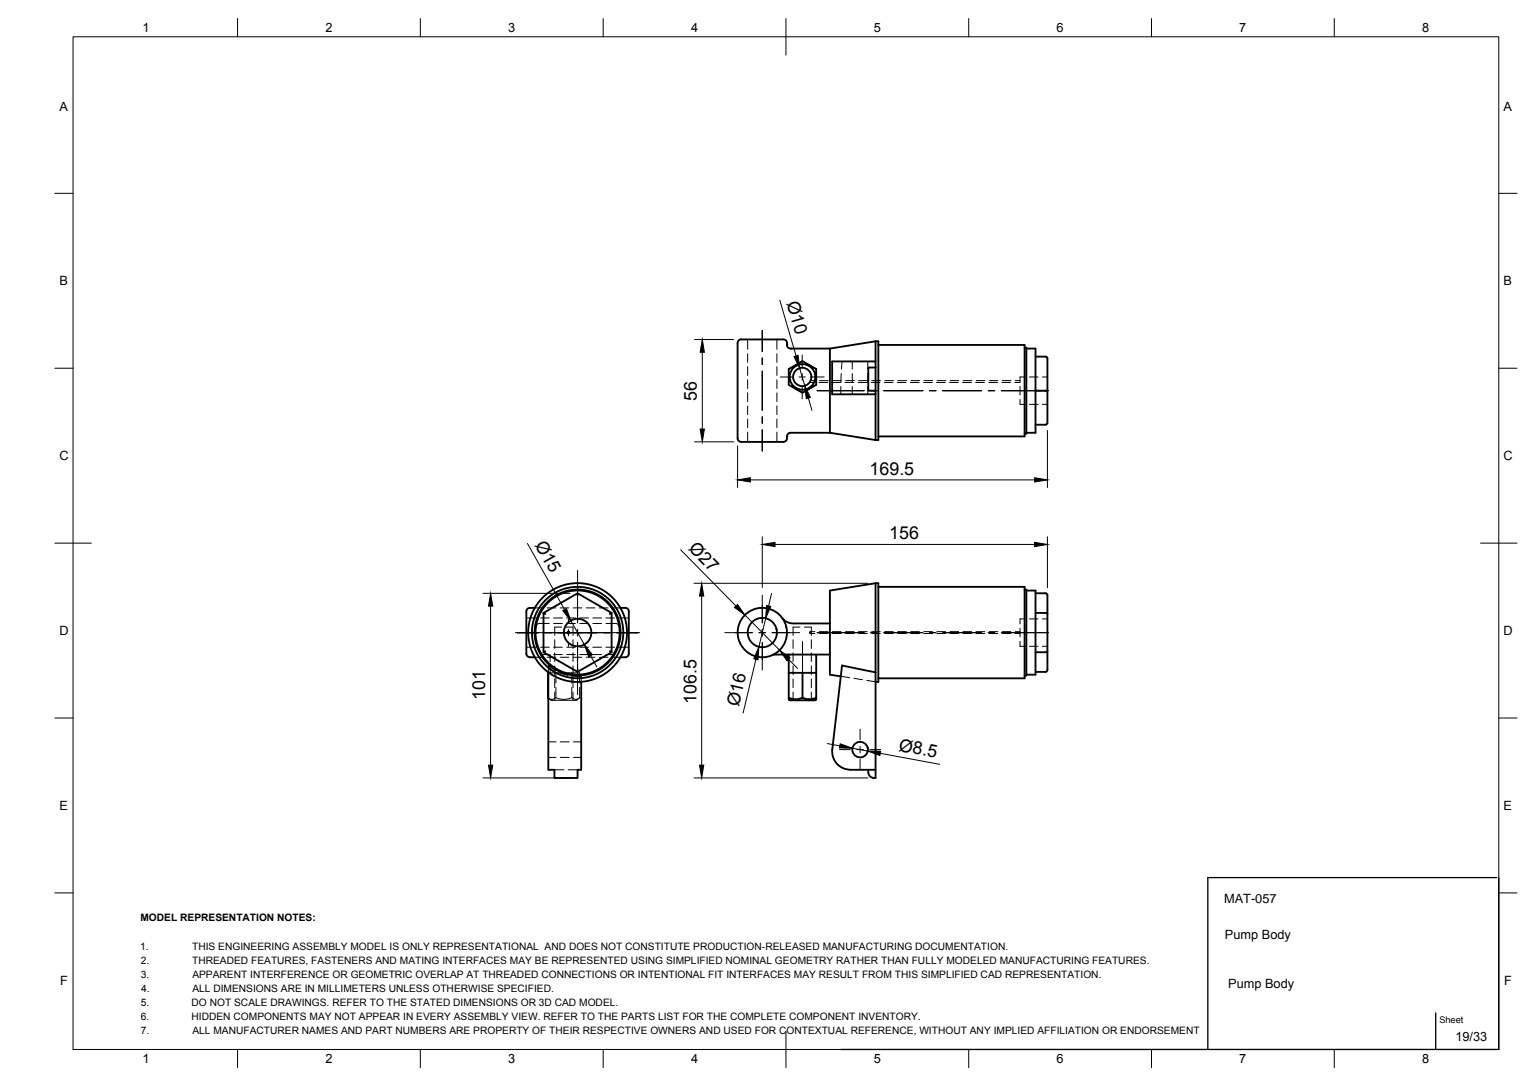
ISO-10303-21;
HEADER;
/* Generated by software containing ST-Developer
 * from STEP Tools, Inc. (www.steptools.com) 
 */

FILE_DESCRIPTION(
/* description */ ('STEP AP214', 'CAx-IF Rec.Pracs.---Representation and Presentation of Product Manufa
cturing Information (PMI)---4.0---2014-10-13'),
/* implementation_level */ '2;1');

FILE_NAME(
/* name */ 'Pump Body.step',
/* time_stamp */ '2026-10-28T23:34:22+01:00',
/* author */ (''),
/* organization */ (''),
/* preprocessor_version */ 'ST-DEVELOPER v20.2',
/* originating_system */ 'Autodesk Translation Framework v15.17.0.0',
/* authorisation */ '');

FILE_SCHEMA (('AP242_MANAGED_MODEL_BASED_3D_ENGINEERING_MIM_LF { 1 0 10303 442 2 1 4 }'));
ENDSEC;

DATA;
#10=MECHANICAL_DESIGN_GEOMETRIC_PRESENTATION_REPRESENTATION('',(#259),#27807);
#35=(
BOUNDED_CURVE()
B_SPLINE_CURVE(2,(#19569,#19570,#19571),.UNSPECIFIED.,.F.,.F.)
B_SPLINE_CURVE_WITH_KNOTS((3,3),(3.35159796330511,5.11240655080017),
 .UNSPECIFIED.)
CURVE()
GEOMETRIC_REPRESENTATION_ITEM()
RATIONAL_B_SPLINE_CURVE((1.02178867577785,1.02219740253536,1.01702175780134))
REPRESENTATION_ITEM('')
);
#213=SHAPE_REPRESENTATION_RELATIONSHIP('SRR','None',#27910,#235);
#235=ADVANCED_BREP_SHAPE_REPRESENTATION('',(#288),#27790);
#259=STYLED_ITEM('',(#28056),#288);
#288=MANIFOLD_SOLID_BREP('Body1',#12035);
#310=(
BOUNDED_SURFACE()
B_SPLINE_SURFACE(3,2,((#20429,#20430,#20431),(#20432,#20433,#20434),(#20435,
#20436,#20437),(#20438,#20439,#20440),(#20441,#20442,#20443),(#20444,#20445,
#20446),(#20447,#20448,#20449),(#20450,#20451,#20452),(#20453,#20454,#20455),
(#20456,#20457,#20458),(#20459,#20460,#20461),(#20462,#20463,#20464),(#20465,
#20466,#20467),(#20468,#20469,#20470)),.UNSPECIFIED.,.F.,.F.,.F.)
B_SPLINE_SURFACE_WITH_KNOTS((4,2,2,2,2,2,4),(3,3),(2.29850860566927E-17,
0.00228352475280831,0.00342528712921246,0.00456704950561661,0.00570881188202075,
0.0068505742584249,0.00913409901123319),(0.,1.),.UNSPECIFIED.)
GEOMETRIC_REPRESENTATION_ITEM()
RATIONAL_B_SPLINE_SURFACE(((1.,0.755928946018453,1.),(1.,0.755919473251654,
1.),(1.,0.756953933195057,1.),(1.,0.759617125008032,1.),(1.,0.760694585385831,
1.),(1.,0.763054974489942,1.),(1.,0.764326129773376,1.),(1.,0.766864760301965,
1.),(1.,0.768132555731698,1.),(1.,0.770457118175421,1.),(1.,0.77151907153067,
1.),(1.,0.773976852479458,1.),(1.,0.774660609303815,1.),(1.,0.773601014837504,
1.)))
REPRESENTATION_ITEM('')
SURFACE()
);
#311=(
BOUNDED_SURFACE()
B_SPLINE_SURFACE(3,2,((#20547,#20548,#20549),(#20550,#20551,#20552),(#20553,
#20554,#20555),(#20556,#20557,#20558),(#20559,#20560,#20561),(#20562,#20563,
#20564),(#20565,#20566,#20567),(#20568,#20569,#20570),(#20571,#20572,#20573),
(#20574,#20575,#20576),(#20577,#20578,#20579),(#20580,#20581,#20582)),
 .UNSPECIFIED.,.F.,.F.,.F.)
B_SPLINE_SURFACE_WITH_KNOTS((4,2,2,2,2,4),(3,3),(-8.67361737988404E-18,
0.0020019127931021,0.00400382558620421,0.00500478198275526,0.00600573837930632,
0.00800765117240843),(0.,1.),.UNSPECIFIED.)
GEOMETRIC_REPRESENTATION_ITEM()
RATIONAL_B_SPLINE_SURFACE(((1.,0.720245417210284,1.),(1.,0.745456109699134,
1.),(1.,0.776939871169668,1.),(1.,0.843085998617067,1.),(1.,0.876043548544159,
1.),(1.,0.919062364122798,1.),(1.,0.932399541573303,1.),(1.,0.955903426154376,
1.),(1.,0.966062375399352,1.),(1.,0.990944979726916,1.),(1.,1.00003808704948,
1.),(1.,1.,1.)))
REPRESENTATION_ITEM('')
SURFACE()
);
#312=(
BOUNDED_SURFACE()
B_SPLINE_SURFACE(3,2,((#20584,#20585,#20586),(#20587,#20588,#20589),(#20590,
#20591,#20592),(#20593,#20594,#20595),(#20596,#20597,#20598),(#20599,#20600,
#20601),(#20602,#20603,#20604),(#20605,#20606,#20607),(#20608,#20609,#20610),
(#20611,#20612,#20613),(#20614,#20615,#20616),(#20617,#20618,#20619),(#20620,
#20621,#20622),(#20623,#20624,#20625),(#20626,#20627,#20628),(#20629,#20630,
#20631),(#20632,#20633,#20634),(#20635,#20636,#20637)),.UNSPECIFIED.,.F.,
 .F.,.F.)
B_SPLINE_SURFACE_WITH_KNOTS((4,2,2,2,2,2,2,2,4),(3,3),(0.0465879948739151,
0.0488019169422094,0.0499088779763565,0.0510158390105036,0.0532297610787979,
0.054336722112945,0.0554436831470922,0.0598715272836807,0.0642993714202692),
(0.,1.),.UNSPECIFIED.)
GEOMETRIC_REPRESENTATION_ITEM()
RATIONAL_B_SPLINE_SURFACE(((1.,0.720245417210284,1.),(1.,0.715430366769561,
1.),(1.,0.711757488391321,1.),(1.,0.708436125845732,1.),(1.,0.707701704610594,
1.),(1.,0.706997400069913,1.),(1.,0.70703042471459,1.),(1.,0.708269366538293,
1.),(1.,0.710603787640094,1.),(1.,0.716102617085572,1.),(1.,0.718267907422322,
1.),(1.,0.723213640275136,1.),(1.,0.726004552476763,1.),(1.,0.741243869654837,
1.),(1.,0.757174433729962,1.),(1.,0.791690080044701,1.),(1.,0.809643404127687,
1.),(1.,0.826358787974886,1.)))
REPRESENTATION_ITEM('')
SURFACE()
);
#313=(
BOUNDED_SURFACE()
B_SPLINE_SURFACE(3,2,((#20719,#20720,#20721),(#20722,#20723,#20724),(#20725,
#20726,#20727),(#20728,#20729,#20730),(#20731,#20732,#20733),(#20734,#20735,
#20736),(#20737,#20738,#20739),(#20740,#20741,#20742),(#20743,#20744,#20745),
(#20746,#20747,#20748),(#20749,#20750,#20751),(#20752,#20753,#20754),(#20755,
#20756,#20757),(#20758,#20759,#20760),(#20761,#20762,#20763),(#20764,#20765,
#20766)),.UNSPECIFIED.,.F.,.F.,.F.)
B_SPLINE_SURFACE_WITH_KNOTS((4,2,2,2,2,2,2,4),(3,3),(0.00572874702066893,
0.00641318489301232,0.00709762276535571,0.00778206063769909,0.00846649851004248,
0.00915093638238587,0.00983537425472925,0.011204249999416),(0.,1.),
 .UNSPECIFIED.)
GEOMETRIC_REPRESENTATION_ITEM()
RATIONAL_B_SPLINE_SURFACE(((1.,0.975506485486288,1.),(1.,0.975513146220073,
1.),(1.,0.973968479244861,1.),(1.,0.968411518445162,1.),(1.,0.964542733059259,
1.),(1.,0.955226889333692,1.),(1.,0.949822152420214,1.),(1.,0.938073995978702,
1.),(1.,0.931687255706716,1.),(1.,0.918003026598242,1.),(1.,0.91068796451963,
1.),(1.,0.895477555573003,1.),(1.,0.887548913896672,1.),(1.,0.862850245396308,
1.),(1.,0.845167627106926,1.),(1.,0.826358787974873,1.)))
REPRESENTATION_ITEM('')
SURFACE()
);
#314=(
BOUNDED_SURFACE()
B_SPLINE_SURFACE(3,2,((#20852,#20853,#20854),(#20855,#20856,#20857),(#20858,
#20859,#20860),(#20861,#20862,#20863),(#20864,#20865,#20866),(#20867,#20868,
#20869),(#20870,#20871,#20872),(#20873,#20874,#20875),(#20876,#20877,#20878),
(#20879,#20880,#20881),(#20882,#20883,#20884),(#20885,#20886,#20887),(#20888,
#20889,#20890),(#20891,#20892,#20893)),.UNSPECIFIED.,.F.,.F.,.F.)
B_SPLINE_SURFACE_WITH_KNOTS((4,2,2,2,2,2,4),(3,3),(2.29850860566927E-17,
0.00228352475280831,0.00342528712921246,0.0045670495056166,0.00570881188202075,
0.00685057425842489,0.00913409901123318),(0.,1.),.UNSPECIFIED.)
GEOMETRIC_REPRESENTATION_ITEM()
RATIONAL_B_SPLINE_SURFACE(((1.,0.755928946018453,1.),(1.,0.755919473252646,
1.),(1.,0.756953933193741,1.),(1.,0.759617125008685,1.),(1.,0.760694585385853,
1.),(1.,0.763054974489921,1.),(1.,0.764326129773228,1.),(1.,0.766864760302113,
1.),(1.,0.76813255573155,1.),(1.,0.77045711817557,1.),(1.,0.77151907153099,
1.),(1.,0.773976852478821,1.),(1.,0.774660609304298,1.),(1.,0.773601014837506,
1.)))
REPRESENTATION_ITEM('')
SURFACE()
);
#315=(
BOUNDED_SURFACE()
B_SPLINE_SURFACE(3,2,((#20970,#20971,#20972),(#20973,#20974,#20975),(#20976,
#20977,#20978),(#20979,#20980,#20981),(#20982,#20983,#20984),(#20985,#20986,
#20987),(#20988,#20989,#20990),(#20991,#20992,#20993),(#20994,#20995,#20996),
(#20997,#20998,#20999),(#21000,#21001,#21002),(#21003,#21004,#21005),(#21006,
#21007,#21008),(#21009,#21010,#21011)),.UNSPECIFIED.,.F.,.F.,.F.)
B_SPLINE_SURFACE_WITH_KNOTS((4,2,2,2,2,2,4),(3,3),(0.0025838157606072,0.0039611177618176,
0.005338419763028,0.0060270707636332,0.0067157217642384,0.0074043727648436,
0.0080930237654488),(0.,1.),.UNSPECIFIED.)
GEOMETRIC_REPRESENTATION_ITEM()
RATIONAL_B_SPLINE_SURFACE(((1.,0.826358787974881,1.),(1.,0.845245405300955,
1.),(1.,0.862939160435579,1.),(1.,0.895803497327567,1.),(1.,0.91098843375652,
1.),(1.,0.931602584770477,1.),(1.,0.938050525530194,1.),(1.,0.949865147477405,
1.),(1.,0.95528172500017,1.),(1.,0.964523416337373,1.),(1.,0.96840980801867,
1.),(1.,0.973963943287705,1.),(1.,0.975504577407296,1.),(1.,0.975506485486285,
1.)))
REPRESENTATION_ITEM('')
SURFACE()
);
#316=(
BOUNDED_SURFACE()
B_SPLINE_SURFACE(3,2,((#21013,#21014,#21015),(#21016,#21017,#21018),(#21019,
#21020,#21021),(#21022,#21023,#21024),(#21025,#21026,#21027),(#21028,#21029,
#21030),(#21031,#21032,#21033),(#21034,#21035,#21036),(#21037,#21038,#21039),
(#21040,#21041,#21042),(#21043,#21044,#21045),(#21046,#21047,#21048)),
 .UNSPECIFIED.,.F.,.F.,.F.)
B_SPLINE_SURFACE_WITH_KNOTS((4,2,2,2,2,4),(3,3),(6.93889390390723E-18,0.00200191279310211,
0.00400382558620421,0.00500478198275526,0.00600573837930631,0.00800765117240842),
(0.,1.),.UNSPECIFIED.)
GEOMETRIC_REPRESENTATION_ITEM()
RATIONAL_B_SPLINE_SURFACE(((1.,0.72024541721028,1.),(1.,0.745456109696734,
1.),(1.,0.776939871172863,1.),(1.,0.843085998613875,1.),(1.,0.876043548543787,
1.),(1.,0.919062364122984,1.),(1.,0.932399541573454,1.),(1.,0.955903426154228,
1.),(1.,0.966062375399276,1.),(1.,0.990944979727062,1.),(1.,1.00003808704937,
1.),(1.,1.,1.)))
REPRESENTATION_ITEM('')
SURFACE()
);
#317=(
BOUNDED_SURFACE()
B_SPLINE_SURFACE(3,2,((#21050,#21051,#21052),(#21053,#21054,#21055),(#21056,
#21057,#21058),(#21059,#21060,#21061),(#21062,#21063,#21064),(#21065,#21066,
#21067),(#21068,#21069,#21070),(#21071,#21072,#21073),(#21074,#21075,#21076),
(#21077,#21078,#21079),(#21080,#21081,#21082),(#21083,#21084,#21085),(#21086,
#21087,#21088),(#21089,#21090,#21091),(#21092,#21093,#21094),(#21095,#21096,
#21097),(#21098,#21099,#21100),(#21101,#21102,#21103),(#21104,#21105,#21106),
(#21107,#21108,#21109),(#21110,#21111,#21112),(#21113,#21114,#21115)),
 .UNSPECIFIED.,.F.,.F.,.F.)
B_SPLINE_SURFACE_WITH_KNOTS((4,2,2,2,2,2,2,2,2,2,4),(3,3),(0.0436602992904701,
0.0480963033926944,0.0491980653433177,0.050299827293941,0.0514015892445644,
0.0525033511951877,0.0547068750964343,0.0558086370470577,0.056910398997681,
0.0591139228989276,0.0613234933874712),(0.,1.00002895629973),
 .UNSPECIFIED.)
GEOMETRIC_REPRESENTATION_ITEM()
RATIONAL_B_SPLINE_SURFACE(((1.,0.826683641938831,1.00001003720082),(1.,
0.809845600472633,1.00001101233558),(1.,0.79184731214926,1.00001205466324),
(1.,0.770216550347386,1.00001330735688),(1.,0.765954721069219,1.00001355417049),
(1.,0.757698677929212,1.00001403229941),(1.,0.753690542776134,1.00001426442094),
(1.,0.745987105952188,1.00001471054699),(1.,0.742291755413244,1.00001492455435),
(1.,0.735294059977715,1.00001532980908),(1.,0.731982797792345,1.00001552157288),
(1.,0.722886163295819,1.00001604838263),(1.,0.71790361921332,1.00001633693471),
(1.,0.712405002570856,1.00001665537389),(1.,0.710901207883209,1.00001674246255),
(1.,0.708608218307941,1.00001687525554),(1.,0.707818554135303,1.00001692098704),
(1.,0.706612720262668,1.00001699082002),(1.,0.707341409991791,1.0000169486197),
(1.,0.711697151558445,1.00001669636739),(1.,0.715335875779425,1.00001648563941),
(1.,0.720277859138149,1.0000161994363)))
REPRESENTATION_ITEM('')
SURFACE()
);
#397=FACE_BOUND('',#2327,.T.);
#398=FACE_BOUND('',#2341,.T.);
#399=FACE_BOUND('',#2345,.T.);
#400=FACE_BOUND('',#2347,.T.);
#401=FACE_BOUND('',#2351,.T.);
#402=FACE_BOUND('',#2353,.T.);
#403=FACE_BOUND('',#2355,.T.);
#404=FACE_BOUND('',#2357,.T.);
#405=FACE_BOUND('',#2365,.T.);
#406=FACE_BOUND('',#2369,.T.);
#407=FACE_BOUND('',#2371,.T.);
#408=FACE_BOUND('',#2390,.T.);
#409=FACE_BOUND('',#2405,.T.);
#588=PLANE('',#13064);
#589=PLANE('',#13066);
#590=PLANE('',#13067);
#591=PLANE('',#13068);
#592=PLANE('',#13069);
#593=PLANE('',#13072);
#594=PLANE('',#13075);
#595=PLANE('',#13076);
#596=PLANE('',#13077);
#597=PLANE('',#13078);
#598=PLANE('',#13079);
#599=PLANE('',#13080);
#600=PLANE('',#13081);
#601=PLANE('',#13082);
#602=PLANE('',#13083);
#603=PLANE('',#13084);
#604=PLANE('',#13085);
#605=PLANE('',#13086);
#606=PLANE('',#13087);
#607=PLANE('',#13088);
#608=PLANE('',#13089);
#609=PLANE('',#13090);
#610=PLANE('',#13091);
#611=PLANE('',#13093);
#612=PLANE('',#13094);
#613=PLANE('',#13096);
#614=PLANE('',#13097);
#615=PLANE('',#13098);
#616=PLANE('',#13099);
#617=PLANE('',#13100);
#618=PLANE('',#13101);
#619=PLANE('',#13102);
#620=PLANE('',#13103);
#621=PLANE('',#13105);
#622=PLANE('',#13107);
#623=PLANE('',#13110);
#624=PLANE('',#13112);
#625=PLANE('',#13114);
#626=PLANE('',#13117);
#627=PLANE('',#13122);
#628=PLANE('',#13123);
#629=PLANE('',#13124);
#630=PLANE('',#13125);
#631=PLANE('',#13126);
#632=PLANE('',#13127);
#633=PLANE('',#13136);
#634=PLANE('',#13137);
#772=ELLIPSE('',#13020,15.2752523147936,9.99999999941178);
#773=ELLIPSE('',#13021,26.5583854086538,10.0763972703331);
#774=ELLIPSE('',#13022,15.2752523156182,9.99999999956869);
#775=ELLIPSE('',#13023,15.2752523175753,10.0000000004984);
#776=ELLIPSE('',#13024,26.4596124709186,10.0015871705796);
#777=ELLIPSE('',#13026,15.2752523173838,10.0000000004154);
#778=ELLIPSE('',#13027,15.2752523164649,9.99999999997215);
#779=ELLIPSE('',#13028,26.5080625328222,10.0382481169211);
#780=ELLIPSE('',#13029,15.2752523159837,9.99999999981764);
#781=ELLIPSE('',#13030,26.3957862331476,9.95339341267837);
#782=ELLIPSE('',#13057,24.57405701212,24.4042521334787);
#783=ELLIPSE('',#13104,15.2752523161817,9.99999999983578);
#784=ELLIPSE('',#13106,15.2752523172107,10.0000000003347);
#785=ELLIPSE('',#13108,15.2752523165152,9.99999999997849);
#786=ELLIPSE('',#13109,15.275252318401,10.0000000008983);
#787=ELLIPSE('',#13111,15.2752523172003,10.0000000003286);
#788=ELLIPSE('',#13113,15.2752523153524,9.99999999942849);
#789=ELLIPSE('',#13115,15.2752523169171,10.0000000001759);
#790=ELLIPSE('',#13116,15.2752523156397,9.99999999956927);
#791=ELLIPSE('',#13118,15.275252316396,9.99999999996106);
#792=ELLIPSE('',#13119,15.2752523165357,10.0000000000049);
#793=ELLIPSE('',#13120,15.2752523165945,10.0000000000236);
#794=ELLIPSE('',#13121,15.2752523165696,10.0000000000157);
#795=ELLIPSE('',#13129,26.271953617607,9.86022278604482);
#796=ELLIPSE('',#13132,26.3549599721588,9.92262765998257);
#797=ELLIPSE('',#13152,1.15470053837393,0.999999999995315);
#798=ELLIPSE('',#13153,1.15470053837848,0.999999999999286);
#799=ELLIPSE('',#13155,1.15470053838003,1.00000000000053);
#800=ELLIPSE('',#13157,1.15470053838039,1.00000000000101);
#801=ELLIPSE('',#13159,1.15470053837954,1.00000000000047);
#802=ELLIPSE('',#13161,1.15470053838034,1.00000000000108);
#829=TOROIDAL_SURFACE('',#12997,11.5,2.);
#830=TOROIDAL_SURFACE('',#13002,11.5,2.);
#877=B_SPLINE_CURVE_WITH_KNOTS('',3,(#19403,#19404,#19405,#19406,#19407,
#19408,#19409,#19410,#19411,#19412,#19413,#19414,#19415,#19416,#19417,#19418,
#19419,#19420),.UNSPECIFIED.,.F.,.F.,(4,2,2,2,2,2,2,2,4),(0.,0.0192470604937845,
0.0384941209875689,0.0593135836604684,0.0801330463333679,0.101727899817301,
0.123322753301234,0.143135709957287,0.162948666613339),.UNSPECIFIED.);
#878=B_SPLINE_CURVE_WITH_KNOTS('',3,(#19424,#19425,#19426,#19427,#19428,
#19429,#19430,#19431,#19432,#19433,#19434,#19435,#19436,#19437,#19438,#19439,
#19440,#19441),.UNSPECIFIED.,.F.,.F.,(4,2,2,2,2,2,2,2,4),(0.162948666613339,
0.181777764507504,0.200606862401668,0.223173739729446,0.245740617057224,
0.267140699938747,0.288540782820269,0.307205908233542,0.325871033646814),
 .UNSPECIFIED.);
#879=B_SPLINE_CURVE_WITH_KNOTS('',3,(#19583,#19584,#19585,#19586),
 .UNSPECIFIED.,.F.,.F.,(4,4),(2.02557768100327E-7,0.0192787307131084),
 .UNSPECIFIED.);
#880=B_SPLINE_CURVE_WITH_KNOTS('',3,(#19591,#19592,#19593,#19594,#19595,
#19596,#19597,#19598,#19599,#19600,#19601,#19602,#19603,#19604,#19605,#19606,
#19607,#19608,#19609,#19610,#19611,#19612),.UNSPECIFIED.,.F.,.F.,(4,3,3,
3,3,3,3,4),(0.0122741017871804,0.0127193579255126,0.013344159318982,0.013690125400826,
0.0139452191691552,0.0145554803714893,0.0151726535547874,0.0156163365512983),
 .UNSPECIFIED.);
#881=B_SPLINE_CURVE_WITH_KNOTS('',3,(#19614,#19615,#19616,#19617,#19618,
#19619,#19620,#19621,#19622,#19623,#19624,#19625,#19626,#19627,#19628,#19629,
#19630,#19631,#19632,#19633,#19634,#19635,#19636,#19637,#19638,#19639,#19640,
#19641,#19642,#19643,#19644,#19645,#19646,#19647,#19648,#19649,#19650,#19651,
#19652,#19653,#19654,#19655,#19656,#19657,#19658,#19659,#19660,#19661,#19662,
#19663,#19664,#19665,#19666,#19667,#19668,#19669,#19670,#19671,#19672,#19673,
#19674,#19675,#19676,#19677,#19678,#19679,#19680),.UNSPECIFIED.,.F.,.F.,
(4,3,3,3,3,3,3,3,3,3,3,3,3,3,3,3,3,3,3,3,3,3,4),(1.38777878078145E-17,0.000359541750743833,
0.000720760360395833,0.000925988989824252,0.00128781683880211,0.00166392003251687,
0.00177264338187088,0.00185197797964849,0.00229111858557702,0.00274334341776006,
0.00322035894802675,0.00360779073578523,0.00370395595929687,0.00429989379062265,
0.00454486050103351,0.00462994494912103,0.00532482870883918,0.00549165268203304,
0.00555593393894519,0.00622533162053515,0.00648192292876935,0.00695499059398613,
0.00740791170339487),.UNSPECIFIED.);
#882=B_SPLINE_CURVE_WITH_KNOTS('',3,(#19684,#19685,#19686,#19687,#19688,
#19689,#19690,#19691,#19692,#19693,#19694,#19695,#19696,#19697,#19698,#19699,
#19700,#19701,#19702,#19703,#19704,#19705,#19706,#19707,#19708,#19709,#19710,
#19711,#19712,#19713,#19714,#19715,#19716,#19717,#19718,#19719,#19720,#19721,
#19722,#19723,#19724,#19725,#19726,#19727,#19728,#19729,#19730,#19731,#19732,
#19733,#19734,#19735,#19736,#19737,#19738,#19739,#19740,#19741,#19742,#19743,
#19744,#19745,#19746,#19747,#19748,#19749,#19750),.UNSPECIFIED.,.F.,.F.,
(4,3,3,3,3,3,3,3,3,3,3,3,3,3,3,3,3,3,3,3,3,3,4),(-1.26412812962169E-5,0.000494289993516549,
0.000916182220770617,0.00158761602821044,0.00184500593803732,0.00190945524103177,
0.00260645980420792,0.00277382965530402,0.00285915079249246,0.00345690366729172,
0.00370265337257072,0.00379909409684229,0.00427723699929272,0.00473898476131605,
0.00517836782884145,0.00556030080710405,0.00563986899627211,0.00601852659233303,
0.00638213905693613,0.00648912452437073,0.00685144713428646,0.00721253712890148,
0.00741794824163741),.UNSPECIFIED.);
#883=B_SPLINE_CURVE_WITH_KNOTS('',3,(#19752,#19753,#19754,#19755,#19756,
#19757),.UNSPECIFIED.,.F.,.F.,(4,2,4),(0.,0.00170403531088726,0.00340807062177452),
 .UNSPECIFIED.);
#884=B_SPLINE_CURVE_WITH_KNOTS('',3,(#19760,#19761,#19762,#19763,#19764,
#19765,#19766,#19767,#19768,#19769,#19770,#19771,#19772,#19773,#19774,#19775),
 .UNSPECIFIED.,.F.,.F.,(4,2,2,2,2,2,2,4),(0.00340807062177452,0.00495591214335585,
0.00650375366493717,0.0080515951865185,0.00959943670809982,0.0111472782296811,
0.0126951197512625,0.0157908027944251),.UNSPECIFIED.);
#885=B_SPLINE_CURVE_WITH_KNOTS('',3,(#19777,#19778,#19779,#19780,#19781,
#19782,#19783,#19784,#19785,#19786,#19787,#19788,#19789,#19790,#19791,#19792,
#19793,#19794,#19795,#19796,#19797,#19798,#19799,#19800,#19801,#19802,#19803,
#19804,#19805,#19806,#19807,#19808,#19809,#19810,#19811,#19812,#19813,#19814,
#19815,#19816,#19817,#19818,#19819,#19820,#19821,#19822,#19823,#19824,#19825,
#19826,#19827,#19828,#19829,#19830,#19831,#19832,#19833,#19834,#19835,#19836,
#19837,#19838,#19839,#19840),.UNSPECIFIED.,.F.,.F.,(4,3,3,3,3,3,3,3,3,3,
3,3,3,3,3,3,3,3,3,3,3,4),(0.,0.000217008353627195,0.00044324659857817,0.000652120823339668,
0.000696799127034378,0.0009320141666111,0.00117457155402921,0.00130424164667934,
0.00137662244777993,0.00162564089691921,0.00188989041240164,0.001956362470019,
0.00203919216218315,0.00242993572455044,0.00260848329335867,0.00268907034510375,
0.00324577551876228,0.00378706053238822,0.00391272494003789,0.0039649107976047,
0.00469438531296503,0.0052169665867171),.UNSPECIFIED.);
#886=B_SPLINE_CURVE_WITH_KNOTS('',3,(#19844,#19845,#19846,#19847,#19848,
#19849,#19850,#19851,#19852,#19853,#19854,#19855,#19856,#19857,#19858,#19859,
#19860,#19861,#19862,#19863,#19864,#19865,#19866,#19867,#19868,#19869,#19870,
#19871,#19872,#19873,#19874,#19875,#19876,#19877,#19878,#19879,#19880,#19881,
#19882,#19883,#19884,#19885,#19886,#19887,#19888,#19889,#19890,#19891,#19892,
#19893,#19894,#19895,#19896,#19897,#19898,#19899,#19900,#19901,#19902,#19903,
#19904,#19905,#19906,#19907,#19908,#19909,#19910,#19911,#19912,#19913),
 .UNSPECIFIED.,.F.,.F.,(4,3,3,3,3,3,3,3,3,3,3,3,3,3,3,3,3,3,3,3,3,3,3,4),
(0.,0.000716363515082861,0.00122272058882501,0.00127670474543072,0.001684939739755,
0.00184333900175369,0.001915057118146,0.0022617033425768,0.00247119369116529,
0.00255340949086129,0.00284871880498323,0.00310811407391612,0.00319176186357658,
0.00345491419006973,0.00370405315221264,0.00375758515241602,0.00383011423629186,
0.00419648947130024,0.00442380729262466,0.00446846660900715,0.00466401696562969,
0.00485470026116451,0.00503802593101401,0.00510681898172244),
 .UNSPECIFIED.);
#887=B_SPLINE_CURVE_WITH_KNOTS('',3,(#19914,#19915,#19916,#19917,#19918,
#19919,#19920,#19921,#19922,#19923,#19924,#19925,#19926,#19927,#19928,#19929,
#19930,#19931),.UNSPECIFIED.,.F.,.F.,(4,2,2,2,2,2,2,2,4),(0.,0.003068525446753,
0.0046027881701295,0.00613705089350601,0.00767131361688251,0.00843844497857076,
0.00920557634025901,0.0107398390636356,0.0122741017870122),
 .UNSPECIFIED.);
#888=B_SPLINE_CURVE_WITH_KNOTS('',3,(#19945,#19946,#19947,#19948,#19949,
#19950,#19951,#19952,#19953,#19954,#19955,#19956,#19957,#19958,#19959,#19960,
#19961,#19962,#19963,#19964,#19965,#19966,#19967,#19968,#19969,#19970,#19971,
#19972,#19973,#19974,#19975,#19976,#19977,#19978,#19979,#19980,#19981,#19982,
#19983,#19984,#19985,#19986,#19987,#19988,#19989,#19990),.UNSPECIFIED.,
 .F.,.F.,(4,3,3,3,3,3,3,3,3,3,3,3,3,3,3,4),(0.,0.00135730202997046,0.00181088490961025,
0.00181523918786338,0.00271632736441538,0.00272329467697279,0.00362176981922051,
0.00363238660702296,0.00452721227402563,0.00454314116852505,0.00525055669087674,
0.00543265472883076,0.00545594202104736,0.0062798042883095,0.00708587073896267,
0.00724353963844092),.UNSPECIFIED.);
#889=B_SPLINE_CURVE_WITH_KNOTS('',3,(#19991,#19992,#19993,#19994,#19995,
#19996,#19997,#19998,#19999,#20000,#20001,#20002,#20003,#20004,#20005,#20006,
#20007,#20008,#20009,#20010,#20011,#20012,#20013,#20014,#20015,#20016,#20017,
#20018,#20019,#20020,#20021,#20022,#20023,#20024,#20025,#20026,#20027,#20028,
#20029,#20030,#20031,#20032,#20033,#20034,#20035,#20036),.UNSPECIFIED.,
 .F.,.F.,(4,3,3,3,3,3,3,3,3,3,3,3,3,3,3,4),(0.,0.000808445975810305,0.00163472102823258,
0.00179462353986192,0.00181800235978474,0.00252819829650182,0.00271101203870707,
0.00272700353967716,0.00362534620384845,0.00363600471956958,0.00453801120277895,
0.00454500589946201,0.00544963568717067,0.00545400707935443,0.00681664400249974,
0.00727200943913927),.UNSPECIFIED.);
#890=B_SPLINE_CURVE_WITH_KNOTS('',3,(#20241,#20242,#20243,#20244),
 .UNSPECIFIED.,.F.,.F.,(4,4),(5.7219584981528E-17,0.00198881562236583),
 .UNSPECIFIED.);
#891=B_SPLINE_CURVE_WITH_KNOTS('',3,(#20248,#20249,#20250,#20251,#20252,
#20253,#20254,#20255,#20256,#20257,#20258,#20259,#20260,#20261,#20262,#20263,
#20264,#20265,#20266,#20267,#20268,#20269,#20270,#20271,#20272,#20273,#20274,
#20275,#20276,#20277,#20278,#20279,#20280,#20281,#20282,#20283,#20284,#20285,
#20286,#20287,#20288,#20289,#20290,#20291,#20292,#20293,#20294,#20295,#20296,
#20297,#20298,#20299,#20300,#20301,#20302,#20303,#20304,#20305,#20306,#20307,
#20308,#20309,#20310,#20311,#20312,#20313,#20314,#20315,#20316,#20317,#20318,
#20319,#20320,#20321,#20322,#20323,#20324,#20325,#20326,#20327,#20328,#20329),
 .UNSPECIFIED.,.F.,.F.,(4,3,3,3,3,3,3,3,3,3,3,3,3,3,3,3,3,3,3,3,3,3,3,3,
3,3,3,4),(1.2719202621569E-16,0.00143589979508649,0.00284404218546533,0.00415362629242205,
0.0042305644511401,0.00504888151365028,0.00519203286552742,0.00527815489686518,
0.00614833446736157,0.00623043943863279,0.00632123327719083,0.00726884601173815,
0.00735976193107753,0.0080560493804554,0.00830725258484352,0.00839384909481171,
0.00982686164286283,0.0103840657310542,0.0104535759650963,0.0114224723041596,
0.0114795275119261,0.0120957876665379,0.012460878877265,0.012503118356934,
0.0135294573324798,0.0145557963080255,0.015608619261337,0.0166145051696864),
 .UNSPECIFIED.);
#892=B_SPLINE_CURVE_WITH_KNOTS('',3,(#20334,#20335,#20336,#20337),
 .UNSPECIFIED.,.F.,.F.,(4,4),(0.,0.00198881562236589),.UNSPECIFIED.);
#893=B_SPLINE_CURVE_WITH_KNOTS('',3,(#20339,#20340,#20341,#20342,#20343,
#20344,#20345,#20346,#20347,#20348,#20349,#20350,#20351,#20352,#20353,#20354,
#20355,#20356,#20357,#20358,#20359,#20360,#20361,#20362,#20363,#20364,#20365,
#20366,#20367,#20368,#20369,#20370,#20371,#20372,#20373,#20374,#20375,#20376,
#20377,#20378,#20379,#20380,#20381,#20382,#20383,#20384,#20385,#20386,#20387,
#20388,#20389,#20390,#20391,#20392,#20393,#20394,#20395,#20396,#20397,#20398,
#20399,#20400,#20401,#20402,#20403,#20404,#20405,#20406,#20407,#20408,#20409,
#20410,#20411,#20412,#20413,#20414,#20415,#20416,#20417,#20418,#20419,#20420,
#20421,#20422,#20423),.UNSPECIFIED.,.F.,.F.,(4,3,3,3,3,3,3,3,3,3,3,3,3,
3,3,3,3,3,3,3,3,3,3,3,3,3,3,3,4),(0.,0.000716458183822177,0.00142634914675041,
0.00205206754060844,0.0020932945390166,0.00296723761715126,0.00308523603842144,
0.00313994180852491,0.00377181010115693,0.00411797980288768,0.00418658907803322,
0.00581684750097351,0.00618890273310859,0.00627988361704989,0.0070571831999972,
0.0072274457512027,0.00732653088655817,0.00795375102207312,0.00826812044930995,
0.00837317815606645,0.00945419362478756,0.0105567220809739,0.0116943447997248,
0.0124737944199864,0.0125597672340995,0.0136064145036077,0.0146658962125278,
0.0157534067466141,0.0167463563121324),.UNSPECIFIED.);
#894=B_SPLINE_CURVE_WITH_KNOTS('',3,(#20471,#20472,#20473,#20474,#20475,
#20476,#20477,#20478,#20479,#20480,#20481,#20482,#20483,#20484,#20485,#20486,
#20487,#20488,#20489,#20490,#20491,#20492,#20493,#20494,#20495,#20496,#20497,
#20498,#20499,#20500,#20501,#20502,#20503,#20504,#20505,#20506,#20507,#20508,
#20509,#20510,#20511,#20512,#20513,#20514,#20515,#20516,#20517,#20518,#20519,
#20520,#20521,#20522,#20523,#20524,#20525,#20526,#20527,#20528,#20529,#20530,
#20531,#20532,#20533,#20534,#20535,#20536,#20537,#20538,#20539,#20540,#20541,
#20542,#20543,#20544,#20545,#20546),.UNSPECIFIED.,.F.,.F.,(4,3,3,3,3,3,
3,3,3,3,3,3,3,3,3,3,3,3,3,3,3,3,3,3,3,4),(2.77988148204925E-13,0.000240598629271839,
0.000486088690534841,0.000739379865323794,0.00086351953650479,0.00109201081567983,
0.00132914312091213,0.00138485296015832,0.00163896000397727,0.00172703907300957,
0.0020510032560785,0.0023836347224887,0.0027322580415582,0.00302289580528531,
0.00335373644476616,0.00345407814601918,0.00382021337536123,0.00392909696477702,
0.00441388534005964,0.00488365632772136,0.00518111721902879,0.00572151392286165,
0.00604463675553361,0.00642122800801736,0.00679034626207549,0.006908156208912),
 .UNSPECIFIED.);
#895=B_SPLINE_CURVE_WITH_KNOTS('',3,(#20640,#20641,#20642,#20643,#20644,
#20645,#20646,#20647,#20648,#20649,#20650,#20651,#20652,#20653,#20654,#20655,
#20656,#20657,#20658,#20659,#20660,#20661,#20662,#20663,#20664,#20665,#20666,
#20667,#20668,#20669,#20670,#20671,#20672,#20673,#20674,#20675,#20676,#20677,
#20678,#20679,#20680,#20681,#20682,#20683,#20684,#20685,#20686,#20687,#20688,
#20689,#20690,#20691,#20692,#20693,#20694,#20695,#20696,#20697,#20698,#20699,
#20700,#20701,#20702,#20703,#20704,#20705,#20706,#20707,#20708,#20709,#20710,
#20711,#20712,#20713,#20714,#20715,#20716,#20717,#20718),.UNSPECIFIED.,
 .F.,.F.,(4,3,3,3,3,3,3,3,3,3,3,3,3,3,3,3,3,3,3,3,3,3,3,3,3,3,4),(0.,7.02681003220256E-5,
0.000143250041041023,0.000221865135200779,0.000253452295756187,0.000331299522547507,
0.000365730675067348,0.000448634730986367,0.000506904591512373,0.00060316276770857,
0.000705610759866986,0.000806172107809853,0.000924817647814786,0.00101380918302463,
0.00117169973492681,0.00130438666521286,0.00150431742405288,0.00171807903281978,
0.00183569921664511,0.00202761836604909,0.00233306873065422,0.00238482361429225,
0.00276944460394528,0.00293994271643501,0.00304142754907356,0.00391372248518797,
0.00405523673209802),.UNSPECIFIED.);
#896=B_SPLINE_CURVE_WITH_KNOTS('',3,(#20773,#20774,#20775,#20776,#20777,
#20778,#20779,#20780,#20781,#20782,#20783,#20784,#20785,#20786,#20787,#20788,
#20789,#20790,#20791,#20792,#20793,#20794,#20795,#20796,#20797,#20798,#20799,
#20800,#20801,#20802,#20803,#20804,#20805,#20806,#20807,#20808,#20809,#20810,
#20811,#20812,#20813,#20814,#20815,#20816,#20817,#20818,#20819,#20820,#20821,
#20822,#20823,#20824,#20825,#20826,#20827,#20828,#20829,#20830,#20831,#20832,
#20833,#20834,#20835,#20836,#20837,#20838,#20839,#20840,#20841,#20842,#20843,
#20844,#20845,#20846,#20847,#20848,#20849,#20850,#20851),.UNSPECIFIED.,
 .F.,.F.,(4,3,3,3,3,3,3,3,3,3,3,3,3,3,3,3,3,3,3,3,3,3,3,3,3,3,4),(0.,0.000574140202871799,
0.00100221889234342,0.00110612621604268,0.0015045731206471,0.00187271135781319,
0.00200443778468684,0.0021955000540258,0.00239948716108467,0.00258607856328849,
0.00272128426511772,0.0028703854494012,0.00300665667703026,0.00311994789192807,
0.0032136798020773,0.00331311536984171,0.00341044074652188,0.00350046922160291,
0.00350776612320204,0.00359009987782602,0.00364838382063052,0.00372718996528856,
0.0037583208462879,0.00382357344841964,0.00388604433371314,0.00394745995154345,
0.00400887556937376),.UNSPECIFIED.);
#897=B_SPLINE_CURVE_WITH_KNOTS('',3,(#20894,#20895,#20896,#20897,#20898,
#20899,#20900,#20901,#20902,#20903,#20904,#20905,#20906,#20907,#20908,#20909,
#20910,#20911,#20912,#20913,#20914,#20915,#20916,#20917,#20918,#20919,#20920,
#20921,#20922,#20923,#20924,#20925,#20926,#20927,#20928,#20929,#20930,#20931,
#20932,#20933,#20934,#20935,#20936,#20937,#20938,#20939,#20940,#20941,#20942,
#20943,#20944,#20945,#20946,#20947,#20948,#20949,#20950,#20951,#20952,#20953,
#20954,#20955,#20956,#20957,#20958,#20959,#20960,#20961,#20962,#20963,#20964,
#20965,#20966,#20967,#20968,#20969),.UNSPECIFIED.,.F.,.F.,(4,3,3,3,3,3,
3,3,3,3,3,3,3,3,3,3,3,3,3,3,3,3,3,3,3,4),(-1.6328271194595E-5,0.000369433773630129,
0.000757274070195943,0.000848560634670326,0.00138981505096866,0.00171344962366214,
0.00201136389971158,0.00249692265816024,0.00296744070560773,0.00333415714234072,
0.00344322760164585,0.00377459389855988,0.00387508241180588,0.00422407835213338,
0.00456272284537112,0.00488624813330148,0.00517300557962956,0.00542751638642631,
0.00551572915222377,0.00575380985097023,0.00598306732204141,0.00603789456862142,
0.00629079704341219,0.00653838705347384,0.00677847963654176,0.00690278355733486),
 .UNSPECIFIED.);
#1099=CYLINDRICAL_SURFACE('',#12995,0.5);
#1100=CYLINDRICAL_SURFACE('',#13007,7.50000000000001);
#1101=CYLINDRICAL_SURFACE('',#13010,5.);
#1102=CYLINDRICAL_SURFACE('',#13013,4.25);
#1103=CYLINDRICAL_SURFACE('',#13016,8.00000000000001);
#1104=CYLINDRICAL_SURFACE('',#13019,10.);
#1105=CYLINDRICAL_SURFACE('',#13025,10.);
#1106=CYLINDRICAL_SURFACE('',#13031,7.50000000000001);
#1107=CYLINDRICAL_SURFACE('',#13039,10.);
#1108=CYLINDRICAL_SURFACE('',#13042,23.);
#1109=CYLINDRICAL_SURFACE('',#13045,23.5);
#1110=CYLINDRICAL_SURFACE('',#13048,25.);
#1111=CYLINDRICAL_SURFACE('',#13051,27.);
#1112=CYLINDRICAL_SURFACE('',#13063,13.5);
#1113=CYLINDRICAL_SURFACE('',#13065,7.75000000000001);
#1114=CYLINDRICAL_SURFACE('',#13128,10.);
#1115=CYLINDRICAL_SURFACE('',#13130,10.);
#1116=CYLINDRICAL_SURFACE('',#13131,10.);
#1117=CYLINDRICAL_SURFACE('',#13133,10.);
#1118=CYLINDRICAL_SURFACE('',#13134,23.);
#1119=CYLINDRICAL_SURFACE('',#13135,23.);
#1120=CYLINDRICAL_SURFACE('',#13138,2.);
#1121=CYLINDRICAL_SURFACE('',#13142,2.);
#1122=CYLINDRICAL_SURFACE('',#13144,2.);
#1123=CYLINDRICAL_SURFACE('',#13146,1.99999999999999);
#1124=CYLINDRICAL_SURFACE('',#13148,2.);
#1125=CYLINDRICAL_SURFACE('',#13151,1.);
#1126=CYLINDRICAL_SURFACE('',#13154,0.999999999999998);
#1127=CYLINDRICAL_SURFACE('',#13156,1.00000000000001);
#1128=CYLINDRICAL_SURFACE('',#13158,0.999999999999998);
#1129=CYLINDRICAL_SURFACE('',#13160,1.00000000000001);
#1130=CYLINDRICAL_SURFACE('',#13162,1.);
#1131=CYLINDRICAL_SURFACE('',#13163,3.00000000000001);
#1563=FACE_OUTER_BOUND('',#2322,.T.);
#1564=FACE_OUTER_BOUND('',#2323,.T.);
#1565=FACE_OUTER_BOUND('',#2324,.T.);
#1566=FACE_OUTER_BOUND('',#2325,.T.);
#1567=FACE_OUTER_BOUND('',#2326,.T.);
#1568=FACE_OUTER_BOUND('',#2328,.T.);
#1569=FACE_OUTER_BOUND('',#2329,.T.);
#1570=FACE_OUTER_BOUND('',#2330,.T.);
#1571=FACE_OUTER_BOUND('',#2331,.T.);
#1572=FACE_OUTER_BOUND('',#2332,.T.);
#1573=FACE_OUTER_BOUND('',#2333,.T.);
#1574=FACE_OUTER_BOUND('',#2334,.T.);
#1575=FACE_OUTER_BOUND('',#2335,.T.);
#1576=FACE_OUTER_BOUND('',#2336,.T.);
#1577=FACE_OUTER_BOUND('',#2337,.T.);
#1578=FACE_OUTER_BOUND('',#2338,.T.);
#1579=FACE_OUTER_BOUND('',#2339,.T.);
#1580=FACE_OUTER_BOUND('',#2340,.T.);
#1581=FACE_OUTER_BOUND('',#2342,.T.);
#1582=FACE_OUTER_BOUND('',#2343,.T.);
#1583=FACE_OUTER_BOUND('',#2344,.T.);
#1584=FACE_OUTER_BOUND('',#2346,.T.);
#1585=FACE_OUTER_BOUND('',#2348,.T.);
#1586=FACE_OUTER_BOUND('',#2349,.T.);
#1587=FACE_OUTER_BOUND('',#2350,.T.);
#1588=FACE_OUTER_BOUND('',#2352,.T.);
#1589=FACE_OUTER_BOUND('',#2354,.T.);
#1590=FACE_OUTER_BOUND('',#2356,.T.);
#1591=FACE_OUTER_BOUND('',#2358,.T.);
#1592=FACE_OUTER_BOUND('',#2359,.T.);
#1593=FACE_OUTER_BOUND('',#2360,.T.);
#1594=FACE_OUTER_BOUND('',#2361,.T.);
#1595=FACE_OUTER_BOUND('',#2362,.T.);
#1596=FACE_OUTER_BOUND('',#2363,.T.);
#1597=FACE_OUTER_BOUND('',#2364,.T.);
#1598=FACE_OUTER_BOUND('',#2366,.T.);
#1599=FACE_OUTER_BOUND('',#2367,.T.);
#1600=FACE_OUTER_BOUND('',#2368,.T.);
#1601=FACE_OUTER_BOUND('',#2370,.T.);
#1602=FACE_OUTER_BOUND('',#2372,.T.);
#1603=FACE_OUTER_BOUND('',#2373,.T.);
#1604=FACE_OUTER_BOUND('',#2374,.T.);
#1605=FACE_OUTER_BOUND('',#2375,.T.);
#1606=FACE_OUTER_BOUND('',#2376,.T.);
#1607=FACE_OUTER_BOUND('',#2377,.T.);
#1608=FACE_OUTER_BOUND('',#2378,.T.);
#1609=FACE_OUTER_BOUND('',#2379,.T.);
#1610=FACE_OUTER_BOUND('',#2380,.T.);
#1611=FACE_OUTER_BOUND('',#2381,.T.);
#1612=FACE_OUTER_BOUND('',#2382,.T.);
#1613=FACE_OUTER_BOUND('',#2383,.T.);
#1614=FACE_OUTER_BOUND('',#2384,.T.);
#1615=FACE_OUTER_BOUND('',#2385,.T.);
#1616=FACE_OUTER_BOUND('',#2386,.T.);
#1617=FACE_OUTER_BOUND('',#2387,.T.);
#1618=FACE_OUTER_BOUND('',#2388,.T.);
#1619=FACE_OUTER_BOUND('',#2389,.T.);
#1620=FACE_OUTER_BOUND('',#2391,.T.);
#1621=FACE_OUTER_BOUND('',#2392,.T.);
#1622=FACE_OUTER_BOUND('',#2393,.T.);
#1623=FACE_OUTER_BOUND('',#2394,.T.);
#1624=FACE_OUTER_BOUND('',#2395,.T.);
#1625=FACE_OUTER_BOUND('',#2396,.T.);
#1626=FACE_OUTER_BOUND('',#2397,.T.);
#1627=FACE_OUTER_BOUND('',#2398,.T.);
#1628=FACE_OUTER_BOUND('',#2399,.T.);
#1629=FACE_OUTER_BOUND('',#2400,.T.);
#1630=FACE_OUTER_BOUND('',#2401,.T.);
#1631=FACE_OUTER_BOUND('',#2402,.T.);
#1632=FACE_OUTER_BOUND('',#2403,.T.);
#1633=FACE_OUTER_BOUND('',#2404,.T.);
#1634=FACE_OUTER_BOUND('',#2406,.T.);
#1635=FACE_OUTER_BOUND('',#2407,.T.);
#1636=FACE_OUTER_BOUND('',#2408,.T.);
#1637=FACE_OUTER_BOUND('',#2409,.T.);
#1638=FACE_OUTER_BOUND('',#2410,.T.);
#1639=FACE_OUTER_BOUND('',#2411,.T.);
#1640=FACE_OUTER_BOUND('',#2412,.T.);
#1641=FACE_OUTER_BOUND('',#2413,.T.);
#1642=FACE_OUTER_BOUND('',#2414,.T.);
#1643=FACE_OUTER_BOUND('',#2415,.T.);
#1644=FACE_OUTER_BOUND('',#2416,.T.);
#1645=FACE_OUTER_BOUND('',#2417,.T.);
#1646=FACE_OUTER_BOUND('',#2418,.T.);
#1647=FACE_OUTER_BOUND('',#2419,.T.);
#1648=FACE_OUTER_BOUND('',#2420,.T.);
#1649=FACE_OUTER_BOUND('',#2421,.T.);
#1650=FACE_OUTER_BOUND('',#2422,.T.);
#1651=FACE_OUTER_BOUND('',#2423,.T.);
#1652=FACE_OUTER_BOUND('',#2424,.T.);
#1653=FACE_OUTER_BOUND('',#2425,.T.);
#2322=EDGE_LOOP('',(#9481,#9482,#9483,#9484,#9485));
#2323=EDGE_LOOP('',(#9486,#9487,#9488,#9489,#9490));
#2324=EDGE_LOOP('',(#9491,#9492,#9493,#9494,#9495));
#2325=EDGE_LOOP('',(#9496,#9497,#9498,#9499));
#2326=EDGE_LOOP('',(#9500,#9501,#9502,#9503));
#2327=EDGE_LOOP('',(#9504,#9505));
#2328=EDGE_LOOP('',(#9506,#9507,#9508,#9509));
#2329=EDGE_LOOP('',(#9510,#9511,#9512,#9513));
#2330=EDGE_LOOP('',(#9514,#9515,#9516,#9517,#9518,#9519,#9520));
#2331=EDGE_LOOP('',(#9521,#9522,#9523,#9524,#9525,#9526,#9527));
#2332=EDGE_LOOP('',(#9528,#9529,#9530,#9531,#9532,#9533,#9534,#9535,#9536));
#2333=EDGE_LOOP('',(#9537,#9538,#9539,#9540));
#2334=EDGE_LOOP('',(#9541,#9542,#9543,#9544));
#2335=EDGE_LOOP('',(#9545,#9546,#9547,#9548));
#2336=EDGE_LOOP('',(#9549,#9550,#9551,#9552));
#2337=EDGE_LOOP('',(#9553,#9554,#9555,#9556,#9557,#9558));
#2338=EDGE_LOOP('',(#9559,#9560,#9561,#9562,#9563,#9564,#9565,#9566,#9567,
#9568,#9569,#9570));
#2339=EDGE_LOOP('',(#9571,#9572,#9573,#9574,#9575,#9576,#9577,#9578,#9579,
#9580,#9581,#9582,#9583,#9584,#9585,#9586,#9587,#9588));
#2340=EDGE_LOOP('',(#9589,#9590,#9591,#9592));
#2341=EDGE_LOOP('',(#9593));
#2342=EDGE_LOOP('',(#9594,#9595,#9596,#9597));
#2343=EDGE_LOOP('',(#9598,#9599,#9600,#9601));
#2344=EDGE_LOOP('',(#9602));
#2345=EDGE_LOOP('',(#9603));
#2346=EDGE_LOOP('',(#9604));
#2347=EDGE_LOOP('',(#9605));
#2348=EDGE_LOOP('',(#9606,#9607,#9608,#9609,#9610));
#2349=EDGE_LOOP('',(#9611,#9612,#9613,#9614));
#2350=EDGE_LOOP('',(#9615));
#2351=EDGE_LOOP('',(#9616));
#2352=EDGE_LOOP('',(#9617));
#2353=EDGE_LOOP('',(#9618));
#2354=EDGE_LOOP('',(#9619));
#2355=EDGE_LOOP('',(#9620));
#2356=EDGE_LOOP('',(#9621));
#2357=EDGE_LOOP('',(#9622,#9623,#9624,#9625,#9626,#9627));
#2358=EDGE_LOOP('',(#9628,#9629,#9630,#9631));
#2359=EDGE_LOOP('',(#9632,#9633,#9634,#9635));
#2360=EDGE_LOOP('',(#9636,#9637,#9638,#9639));
#2361=EDGE_LOOP('',(#9640,#9641,#9642,#9643));
#2362=EDGE_LOOP('',(#9644,#9645,#9646,#9647));
#2363=EDGE_LOOP('',(#9648,#9649,#9650,#9651));
#2364=EDGE_LOOP('',(#9652,#9653,#9654,#9655,#9656,#9657));
#2365=EDGE_LOOP('',(#9658));
#2366=EDGE_LOOP('',(#9659,#9660,#9661,#9662,#9663,#9664,#9665,#9666));
#2367=EDGE_LOOP('',(#9667,#9668,#9669,#9670,#9671,#9672,#9673,#9674));
#2368=EDGE_LOOP('',(#9675,#9676,#9677,#9678,#9679));
#2369=EDGE_LOOP('',(#9680));
#2370=EDGE_LOOP('',(#9681,#9682,#9683,#9684,#9685));
#2371=EDGE_LOOP('',(#9686));
#2372=EDGE_LOOP('',(#9687,#9688,#9689,#9690));
#2373=EDGE_LOOP('',(#9691,#9692,#9693,#9694,#9695));
#2374=EDGE_LOOP('',(#9696,#9697,#9698,#9699));
#2375=EDGE_LOOP('',(#9700,#9701,#9702,#9703,#9704));
#2376=EDGE_LOOP('',(#9705,#9706,#9707,#9708));
#2377=EDGE_LOOP('',(#9709,#9710,#9711));
#2378=EDGE_LOOP('',(#9712,#9713,#9714));
#2379=EDGE_LOOP('',(#9715,#9716,#9717));
#2380=EDGE_LOOP('',(#9718,#9719,#9720));
#2381=EDGE_LOOP('',(#9721,#9722,#9723));
#2382=EDGE_LOOP('',(#9724,#9725,#9726));
#2383=EDGE_LOOP('',(#9727,#9728,#9729,#9730,#9731,#9732,#9733));
#2384=EDGE_LOOP('',(#9734,#9735,#9736,#9737,#9738,#9739,#9740));
#2385=EDGE_LOOP('',(#9741,#9742,#9743,#9744,#9745,#9746,#9747));
#2386=EDGE_LOOP('',(#9748,#9749,#9750,#9751,#9752,#9753,#9754));
#2387=EDGE_LOOP('',(#9755,#9756,#9757,#9758,#9759,#9760,#9761));
#2388=EDGE_LOOP('',(#9762,#9763,#9764,#9765,#9766,#9767,#9768));
#2389=EDGE_LOOP('',(#9769,#9770,#9771,#9772,#9773,#9774));
#2390=EDGE_LOOP('',(#9775));
#2391=EDGE_LOOP('',(#9776,#9777,#9778));
#2392=EDGE_LOOP('',(#9779,#9780,#9781));
#2393=EDGE_LOOP('',(#9782,#9783,#9784));
#2394=EDGE_LOOP('',(#9785,#9786,#9787));
#2395=EDGE_LOOP('',(#9788,#9789,#9790));
#2396=EDGE_LOOP('',(#9791,#9792,#9793));
#2397=EDGE_LOOP('',(#9794,#9795,#9796,#9797,#9798,#9799,#9800));
#2398=EDGE_LOOP('',(#9801,#9802,#9803,#9804,#9805,#9806,#9807));
#2399=EDGE_LOOP('',(#9808,#9809,#9810,#9811,#9812,#9813,#9814));
#2400=EDGE_LOOP('',(#9815,#9816,#9817,#9818,#9819,#9820,#9821));
#2401=EDGE_LOOP('',(#9822,#9823,#9824,#9825,#9826));
#2402=EDGE_LOOP('',(#9827,#9828,#9829,#9830,#9831));
#2403=EDGE_LOOP('',(#9832));
#2404=EDGE_LOOP('',(#9833));
#2405=EDGE_LOOP('',(#9834));
#2406=EDGE_LOOP('',(#9835,#9836,#9837,#9838));
#2407=EDGE_LOOP('',(#9839,#9840,#9841,#9842));
#2408=EDGE_LOOP('',(#9843,#9844,#9845));
#2409=EDGE_LOOP('',(#9846,#9847,#9848,#9849,#9850));
#2410=EDGE_LOOP('',(#9851,#9852,#9853,#9854));
#2411=EDGE_LOOP('',(#9855,#9856,#9857,#9858));
#2412=EDGE_LOOP('',(#9859,#9860,#9861,#9862));
#2413=EDGE_LOOP('',(#9863,#9864,#9865,#9866));
#2414=EDGE_LOOP('',(#9867,#9868,#9869,#9870));
#2415=EDGE_LOOP('',(#9871,#9872,#9873,#9874));
#2416=EDGE_LOOP('',(#9875,#9876,#9877,#9878));
#2417=EDGE_LOOP('',(#9879,#9880,#9881));
#2418=EDGE_LOOP('',(#9882,#9883,#9884,#9885,#9886));
#2419=EDGE_LOOP('',(#9887,#9888,#9889,#9890));
#2420=EDGE_LOOP('',(#9891,#9892,#9893,#9894));
#2421=EDGE_LOOP('',(#9895,#9896,#9897,#9898));
#2422=EDGE_LOOP('',(#9899,#9900,#9901,#9902));
#2423=EDGE_LOOP('',(#9903,#9904,#9905,#9906));
#2424=EDGE_LOOP('',(#9907,#9908,#9909,#9910));
#2425=EDGE_LOOP('',(#9911,#9912,#9913,#9914));
#3160=LINE('',#19422,#3980);
#3161=LINE('',#19462,#3981);
#3162=LINE('',#19468,#3982);
#3163=LINE('',#19474,#3983);
#3164=LINE('',#19480,#3984);
#3165=LINE('',#19489,#3985);
#3166=LINE('',#19495,#3986);
#3167=LINE('',#19504,#3987);
#3168=LINE('',#19511,#3988);
#3169=LINE('',#19516,#3989);
#3170=LINE('',#19533,#3990);
#3171=LINE('',#19536,#3991);
#3172=LINE('',#19541,#3992);
#3173=LINE('',#19547,#3993);
#3174=LINE('',#19553,#3994);
#3175=LINE('',#19559,#3995);
#3176=LINE('',#19573,#3996);
#3177=LINE('',#19589,#3997);
#3178=LINE('',#19682,#3998);
#3179=LINE('',#19758,#3999);
#3180=LINE('',#19842,#4000);
#3181=LINE('',#19935,#4001);
#3182=LINE('',#19937,#4002);
#3183=LINE('',#19939,#4003);
#3184=LINE('',#19940,#4004);
#3185=LINE('',#19944,#4005);
#3186=LINE('',#20040,#4006);
#3187=LINE('',#20041,#4007);
#3188=LINE('',#20042,#4008);
#3189=LINE('',#20057,#4009);
#3190=LINE('',#20059,#4010);
#3191=LINE('',#20061,#4011);
#3192=LINE('',#20063,#4012);
#3193=LINE('',#20065,#4013);
#3194=LINE('',#20066,#4014);
#3195=LINE('',#20069,#4015);
#3196=LINE('',#20071,#4016);
#3197=LINE('',#20072,#4017);
#3198=LINE('',#20075,#4018);
#3199=LINE('',#20076,#4019);
#3200=LINE('',#20079,#4020);
#3201=LINE('',#20080,#4021);
#3202=LINE('',#20083,#4022);
#3203=LINE('',#20084,#4023);
#3204=LINE('',#20087,#4024);
#3205=LINE('',#20088,#4025);
#3206=LINE('',#20090,#4026);
#3207=LINE('',#20094,#4027);
#3208=LINE('',#20096,#4028);
#3209=LINE('',#20098,#4029);
#3210=LINE('',#20100,#4030);
#3211=LINE('',#20102,#4031);
#3212=LINE('',#20103,#4032);
#3213=LINE('',#20107,#4033);
#3214=LINE('',#20109,#4034);
#3215=LINE('',#20111,#4035);
#3216=LINE('',#20113,#4036);
#3217=LINE('',#20114,#4037);
#3218=LINE('',#20116,#4038);
#3219=LINE('',#20117,#4039);
#3220=LINE('',#20119,#4040);
#3221=LINE('',#20121,#4041);
#3222=LINE('',#20123,#4042);
#3223=LINE('',#20124,#4043);
#3224=LINE('',#20125,#4044);
#3225=LINE('',#20127,#4045);
#3226=LINE('',#20129,#4046);
#3227=LINE('',#20133,#4047);
#3228=LINE('',#20136,#4048);
#3229=LINE('',#20139,#4049);
#3230=LINE('',#20140,#4050);
#3231=LINE('',#20143,#4051);
#3232=LINE('',#20146,#4052);
#3233=LINE('',#20149,#4053);
#3234=LINE('',#20150,#4054);
#3235=LINE('',#20153,#4055);
#3236=LINE('',#20154,#4056);
#3237=LINE('',#20157,#4057);
#3238=LINE('',#20158,#4058);
#3239=LINE('',#20161,#4059);
#3240=LINE('',#20162,#4060);
#3241=LINE('',#20165,#4061);
#3242=LINE('',#20166,#4062);
#3243=LINE('',#20169,#4063);
#3244=LINE('',#20170,#4064);
#3245=LINE('',#20173,#4065);
#3246=LINE('',#20176,#4066);
#3247=LINE('',#20177,#4067);
#3248=LINE('',#20180,#4068);
#3249=LINE('',#20182,#4069);
#3250=LINE('',#20187,#4070);
#3251=LINE('',#20190,#4071);
#3252=LINE('',#20194,#4072);
#3253=LINE('',#20196,#4073);
#3254=LINE('',#20199,#4074);
#3255=LINE('',#20202,#4075);
#3256=LINE('',#20207,#4076);
#3257=LINE('',#20217,#4077);
#3258=LINE('',#20219,#4078);
#3259=LINE('',#20222,#4079);
#3260=LINE('',#20223,#4080);
#3261=LINE('',#20226,#4081);
#3262=LINE('',#20227,#4082);
#3263=LINE('',#20229,#4083);
#3264=LINE('',#20231,#4084);
#3265=LINE('',#20245,#4085);
#3266=LINE('',#20247,#4086);
#3267=LINE('',#20332,#4087);
#3268=LINE('',#20424,#4088);
#3980=VECTOR('',#15534,0.5);
#3981=VECTOR('',#15561,7.50000000000001);
#3982=VECTOR('',#15568,5.00000000000001);
#3983=VECTOR('',#15575,4.25);
#3984=VECTOR('',#15582,8.00000000000001);
#3985=VECTOR('',#15591,1000.);
#3986=VECTOR('',#15596,1000.);
#3987=VECTOR('',#15605,1000.);
#3988=VECTOR('',#15612,1000.);
#3989=VECTOR('',#15617,7.50000000000001);
#3990=VECTOR('',#15634,1000.);
#3991=VECTOR('',#15637,1000.);
#3992=VECTOR('',#15642,23.);
#3993=VECTOR('',#15649,23.5);
#3994=VECTOR('',#15656,25.);
#3995=VECTOR('',#15663,27.);
#3996=VECTOR('',#15674,27.);
#3997=VECTOR('',#15687,13.5);
#3998=VECTOR('',#15688,1000.);
#3999=VECTOR('',#15689,13.5);
#4000=VECTOR('',#15690,1000.);
#4001=VECTOR('',#15693,1000.);
#4002=VECTOR('',#15694,1000.);
#4003=VECTOR('',#15695,1000.);
#4004=VECTOR('',#15696,1000.);
#4005=VECTOR('',#15699,1000.);
#4006=VECTOR('',#15702,1000.);
#4007=VECTOR('',#15703,1000.);
#4008=VECTOR('',#15704,1000.);
#4009=VECTOR('',#15729,1000.);
#4010=VECTOR('',#15730,1000.);
#4011=VECTOR('',#15731,1000.);
#4012=VECTOR('',#15732,1000.);
#4013=VECTOR('',#15733,1000.);
#4014=VECTOR('',#15734,1000.);
#4015=VECTOR('',#15737,1000.);
#4016=VECTOR('',#15738,1000.);
#4017=VECTOR('',#15739,1000.);
#4018=VECTOR('',#15742,1000.);
#4019=VECTOR('',#15743,1000.);
#4020=VECTOR('',#15746,1000.);
#4021=VECTOR('',#15747,1000.);
#4022=VECTOR('',#15750,1000.);
#4023=VECTOR('',#15751,1000.);
#4024=VECTOR('',#15754,1000.);
#4025=VECTOR('',#15755,1000.);
#4026=VECTOR('',#15758,1000.);
#4027=VECTOR('',#15761,1000.);
#4028=VECTOR('',#15762,1000.);
#4029=VECTOR('',#15763,1000.);
#4030=VECTOR('',#15764,1000.);
#4031=VECTOR('',#15765,1000.);
#4032=VECTOR('',#15766,1000.);
#4033=VECTOR('',#15769,1000.);
#4034=VECTOR('',#15770,1000.);
#4035=VECTOR('',#15771,1000.);
#4036=VECTOR('',#15772,10.);
#4037=VECTOR('',#15773,10.);
#4038=VECTOR('',#15774,10.);
#4039=VECTOR('',#15775,10.);
#4040=VECTOR('',#15778,1000.);
#4041=VECTOR('',#15779,1000.);
#4042=VECTOR('',#15780,1000.);
#4043=VECTOR('',#15781,1000.);
#4044=VECTOR('',#15782,1000.);
#4045=VECTOR('',#15785,1000.);
#4046=VECTOR('',#15788,1000.);
#4047=VECTOR('',#15793,1000.);
#4048=VECTOR('',#15796,1000.);
#4049=VECTOR('',#15799,1000.);
#4050=VECTOR('',#15800,1000.);
#4051=VECTOR('',#15803,1000.);
#4052=VECTOR('',#15808,1000.);
#4053=VECTOR('',#15811,1000.);
#4054=VECTOR('',#15812,1000.);
#4055=VECTOR('',#15815,1000.);
#4056=VECTOR('',#15816,1000.);
#4057=VECTOR('',#15819,1000.);
#4058=VECTOR('',#15820,1000.);
#4059=VECTOR('',#15823,1000.);
#4060=VECTOR('',#15824,1000.);
#4061=VECTOR('',#15827,1000.);
#4062=VECTOR('',#15828,1000.);
#4063=VECTOR('',#15831,1000.);
#4064=VECTOR('',#15832,1000.);
#4065=VECTOR('',#15835,1000.);
#4066=VECTOR('',#15838,1000.);
#4067=VECTOR('',#15839,1000.);
#4068=VECTOR('',#15842,1000.);
#4069=VECTOR('',#15843,1000.);
#4070=VECTOR('',#15848,1000.);
#4071=VECTOR('',#15851,1000.);
#4072=VECTOR('',#15856,1000.);
#4073=VECTOR('',#15859,1000.);
#4074=VECTOR('',#15862,1000.);
#4075=VECTOR('',#15865,1000.);
#4076=VECTOR('',#15870,1000.);
#4077=VECTOR('',#15885,1000.);
#4078=VECTOR('',#15888,1000.);
#4079=VECTOR('',#15891,1000.);
#4080=VECTOR('',#15892,1000.);
#4081=VECTOR('',#15895,1000.);
#4082=VECTOR('',#15896,1000.);
#4083=VECTOR('',#15899,1000.);
#4084=VECTOR('',#15902,1000.);
#4085=VECTOR('',#15917,1000.);
#4086=VECTOR('',#15918,1000.);
#4087=VECTOR('',#15921,1000.);
#4088=VECTOR('',#15922,1000.);
#4735=CIRCLE('',#12996,0.5);
#4736=CIRCLE('',#12998,11.5);
#4737=CIRCLE('',#12999,2.);
#4738=CIRCLE('',#13000,13.5);
#4739=CIRCLE('',#13001,13.5);
#4740=CIRCLE('',#13003,13.5);
#4741=CIRCLE('',#13004,13.5);
#4742=CIRCLE('',#13005,2.);
#4743=CIRCLE('',#13006,11.5);
#4744=CIRCLE('',#13008,7.50000000000001);
#4745=CIRCLE('',#13009,7.50000000000001);
#4746=CIRCLE('',#13011,5.);
#4747=CIRCLE('',#13012,5.);
#4748=CIRCLE('',#13014,4.25);
#4749=CIRCLE('',#13015,4.25);
#4750=CIRCLE('',#13017,8.00000000000001);
#4751=CIRCLE('',#13018,8.00000000000001);
#4752=CIRCLE('',#13032,7.50000000000001);
#4753=CIRCLE('',#13033,7.50000000000001);
#4754=CIRCLE('',#13034,7.50000000000001);
#4755=CIRCLE('',#13035,7.50000000000001);
#4756=CIRCLE('',#13036,7.50000000000001);
#4757=CIRCLE('',#13037,7.50000000000001);
#4758=CIRCLE('',#13038,7.50000000000001);
#4759=CIRCLE('',#13040,10.);
#4760=CIRCLE('',#13041,9.99999999999999);
#4761=CIRCLE('',#13043,23.);
#4762=CIRCLE('',#13044,23.);
#4763=CIRCLE('',#13046,23.5);
#4764=CIRCLE('',#13047,23.5);
#4765=CIRCLE('',#13049,25.);
#4766=CIRCLE('',#13050,25.);
#4767=CIRCLE('',#13052,27.);
#4768=CIRCLE('',#13053,27.);
#4769=CIRCLE('',#13054,27.);
#4770=CIRCLE('',#13055,27.);
#4771=CIRCLE('',#13058,23.);
#4772=CIRCLE('',#13059,23.);
#4773=CIRCLE('',#13060,23.);
#4774=CIRCLE('',#13061,23.);
#4775=CIRCLE('',#13062,23.);
#4776=CIRCLE('',#13070,2.);
#4777=CIRCLE('',#13071,2.);
#4778=CIRCLE('',#13073,2.);
#4779=CIRCLE('',#13074,2.);
#4780=CIRCLE('',#13092,3.00000000000001);
#4781=CIRCLE('',#13095,2.99999999999999);
#4782=CIRCLE('',#13139,2.);
#4783=CIRCLE('',#13140,2.00000000000002);
#4784=CIRCLE('',#13141,2.00000000000001);
#4785=CIRCLE('',#13143,1.99999999999999);
#4786=CIRCLE('',#13145,2.);
#4787=CIRCLE('',#13147,1.99999999999999);
#4788=CIRCLE('',#13149,1.99999999999999);
#4789=CIRCLE('',#13150,2.00000000000002);
#5564=VERTEX_POINT('',#19401);
#5565=VERTEX_POINT('',#19402);
#5566=VERTEX_POINT('',#19421);
#5567=VERTEX_POINT('',#19443);
#5568=VERTEX_POINT('',#19445);
#5569=VERTEX_POINT('',#19447);
#5570=VERTEX_POINT('',#19451);
#5571=VERTEX_POINT('',#19452);
#5572=VERTEX_POINT('',#19455);
#5573=VERTEX_POINT('',#19459);
#5574=VERTEX_POINT('',#19461);
#5575=VERTEX_POINT('',#19465);
#5576=VERTEX_POINT('',#19467);
#5577=VERTEX_POINT('',#19471);
#5578=VERTEX_POINT('',#19473);
#5579=VERTEX_POINT('',#19477);
#5580=VERTEX_POINT('',#19479);
#5581=VERTEX_POINT('',#19483);
#5582=VERTEX_POINT('',#19484);
#5583=VERTEX_POINT('',#19486);
#5584=VERTEX_POINT('',#19488);
#5585=VERTEX_POINT('',#19490);
#5586=VERTEX_POINT('',#19492);
#5587=VERTEX_POINT('',#19494);
#5588=VERTEX_POINT('',#19498);
#5589=VERTEX_POINT('',#19499);
#5590=VERTEX_POINT('',#19501);
#5591=VERTEX_POINT('',#19503);
#5592=VERTEX_POINT('',#19505);
#5593=VERTEX_POINT('',#19507);
#5594=VERTEX_POINT('',#19509);
#5595=VERTEX_POINT('',#19513);
#5596=VERTEX_POINT('',#19515);
#5597=VERTEX_POINT('',#19517);
#5598=VERTEX_POINT('',#19519);
#5599=VERTEX_POINT('',#19521);
#5600=VERTEX_POINT('',#19523);
#5601=VERTEX_POINT('',#19525);
#5602=VERTEX_POINT('',#19529);
#5603=VERTEX_POINT('',#19530);
#5604=VERTEX_POINT('',#19532);
#5605=VERTEX_POINT('',#19534);
#5606=VERTEX_POINT('',#19538);
#5607=VERTEX_POINT('',#19540);
#5608=VERTEX_POINT('',#19544);
#5609=VERTEX_POINT('',#19546);
#5610=VERTEX_POINT('',#19550);
#5611=VERTEX_POINT('',#19552);
#5612=VERTEX_POINT('',#19556);
#5613=VERTEX_POINT('',#19558);
#5614=VERTEX_POINT('',#19560);
#5615=VERTEX_POINT('',#19562);
#5616=VERTEX_POINT('',#19566);
#5617=VERTEX_POINT('',#19567);
#5618=VERTEX_POINT('',#19572);
#5619=VERTEX_POINT('',#19574);
#5620=VERTEX_POINT('',#19576);
#5621=VERTEX_POINT('',#19578);
#5622=VERTEX_POINT('',#19580);
#5623=VERTEX_POINT('',#19588);
#5624=VERTEX_POINT('',#19590);
#5625=VERTEX_POINT('',#19613);
#5626=VERTEX_POINT('',#19681);
#5627=VERTEX_POINT('',#19683);
#5628=VERTEX_POINT('',#19751);
#5629=VERTEX_POINT('',#19759);
#5630=VERTEX_POINT('',#19776);
#5631=VERTEX_POINT('',#19841);
#5632=VERTEX_POINT('',#19843);
#5633=VERTEX_POINT('',#19933);
#5634=VERTEX_POINT('',#19934);
#5635=VERTEX_POINT('',#19936);
#5636=VERTEX_POINT('',#19938);
#5637=VERTEX_POINT('',#19942);
#5638=VERTEX_POINT('',#19943);
#5639=VERTEX_POINT('',#20038);
#5640=VERTEX_POINT('',#20039);
#5641=VERTEX_POINT('',#20055);
#5642=VERTEX_POINT('',#20056);
#5643=VERTEX_POINT('',#20058);
#5644=VERTEX_POINT('',#20060);
#5645=VERTEX_POINT('',#20062);
#5646=VERTEX_POINT('',#20064);
#5647=VERTEX_POINT('',#20068);
#5648=VERTEX_POINT('',#20070);
#5649=VERTEX_POINT('',#20074);
#5650=VERTEX_POINT('',#20078);
#5651=VERTEX_POINT('',#20082);
#5652=VERTEX_POINT('',#20086);
#5653=VERTEX_POINT('',#20092);
#5654=VERTEX_POINT('',#20093);
#5655=VERTEX_POINT('',#20095);
#5656=VERTEX_POINT('',#20097);
#5657=VERTEX_POINT('',#20099);
#5658=VERTEX_POINT('',#20101);
#5659=VERTEX_POINT('',#20105);
#5660=VERTEX_POINT('',#20106);
#5661=VERTEX_POINT('',#20108);
#5662=VERTEX_POINT('',#20110);
#5663=VERTEX_POINT('',#20112);
#5664=VERTEX_POINT('',#20115);
#5665=VERTEX_POINT('',#20120);
#5666=VERTEX_POINT('',#20122);
#5667=VERTEX_POINT('',#20132);
#5668=VERTEX_POINT('',#20134);
#5669=VERTEX_POINT('',#20138);
#5670=VERTEX_POINT('',#20142);
#5671=VERTEX_POINT('',#20148);
#5672=VERTEX_POINT('',#20152);
#5673=VERTEX_POINT('',#20156);
#5674=VERTEX_POINT('',#20160);
#5675=VERTEX_POINT('',#20164);
#5676=VERTEX_POINT('',#20168);
#5677=VERTEX_POINT('',#20172);
#5678=VERTEX_POINT('',#20174);
#5679=VERTEX_POINT('',#20179);
#5680=VERTEX_POINT('',#20181);
#5681=VERTEX_POINT('',#20185);
#5682=VERTEX_POINT('',#20186);
#5683=VERTEX_POINT('',#20189);
#5684=VERTEX_POINT('',#20193);
#5685=VERTEX_POINT('',#20198);
#5686=VERTEX_POINT('',#20200);
#5687=VERTEX_POINT('',#20204);
#5688=VERTEX_POINT('',#20206);
#5689=VERTEX_POINT('',#20210);
#5690=VERTEX_POINT('',#20213);
#5691=VERTEX_POINT('',#20221);
#5692=VERTEX_POINT('',#20225);
#5693=VERTEX_POINT('',#20239);
#5694=VERTEX_POINT('',#20240);
#5695=VERTEX_POINT('',#20246);
#5696=VERTEX_POINT('',#20331);
#5697=VERTEX_POINT('',#20333);
#5698=VERTEX_POINT('',#20338);
#6953=EDGE_CURVE('',#5564,#5565,#877,.T.);
#6954=EDGE_CURVE('',#5565,#5566,#3160,.T.);
#6955=EDGE_CURVE('',#5566,#5566,#4735,.T.);
#6956=EDGE_CURVE('',#5565,#5564,#878,.T.);
#6957=EDGE_CURVE('',#5567,#5567,#4736,.T.);
#6958=EDGE_CURVE('',#5567,#5568,#4737,.T.);
#6959=EDGE_CURVE('',#5569,#5568,#4738,.T.);
#6960=EDGE_CURVE('',#5568,#5569,#4739,.T.);
#6961=EDGE_CURVE('',#5570,#5571,#4740,.T.);
#6962=EDGE_CURVE('',#5571,#5570,#4741,.T.);
#6963=EDGE_CURVE('',#5571,#5572,#4742,.T.);
#6964=EDGE_CURVE('',#5572,#5572,#4743,.T.);
#6965=EDGE_CURVE('',#5573,#5573,#4744,.T.);
#6966=EDGE_CURVE('',#5573,#5574,#3161,.T.);
#6967=EDGE_CURVE('',#5574,#5574,#4745,.T.);
#6968=EDGE_CURVE('',#5575,#5575,#4746,.T.);
#6969=EDGE_CURVE('',#5575,#5576,#3162,.T.);
#6970=EDGE_CURVE('',#5576,#5576,#4747,.T.);
#6971=EDGE_CURVE('',#5577,#5577,#4748,.T.);
#6972=EDGE_CURVE('',#5577,#5578,#3163,.T.);
#6973=EDGE_CURVE('',#5578,#5578,#4749,.T.);
#6974=EDGE_CURVE('',#5579,#5579,#4750,.T.);
#6975=EDGE_CURVE('',#5579,#5580,#3164,.T.);
#6976=EDGE_CURVE('',#5580,#5580,#4751,.T.);
#6977=EDGE_CURVE('',#5581,#5582,#772,.T.);
#6978=EDGE_CURVE('',#5583,#5581,#773,.T.);
#6979=EDGE_CURVE('',#5584,#5583,#3165,.T.);
#6980=EDGE_CURVE('',#5585,#5584,#774,.T.);
#6981=EDGE_CURVE('',#5586,#5585,#775,.T.);
#6982=EDGE_CURVE('',#5587,#5586,#3166,.T.);
#6983=EDGE_CURVE('',#5587,#5582,#776,.T.);
#6984=EDGE_CURVE('',#5588,#5589,#777,.T.);
#6985=EDGE_CURVE('',#5590,#5588,#778,.T.);
#6986=EDGE_CURVE('',#5591,#5590,#3167,.T.);
#6987=EDGE_CURVE('',#5592,#5591,#779,.T.);
#6988=EDGE_CURVE('',#5593,#5592,#780,.T.);
#6989=EDGE_CURVE('',#5593,#5594,#781,.T.);
#6990=EDGE_CURVE('',#5589,#5594,#3168,.T.);
#6991=EDGE_CURVE('',#5595,#5595,#4752,.T.);
#6992=EDGE_CURVE('',#5595,#5596,#3169,.T.);
#6993=EDGE_CURVE('',#5597,#5596,#4753,.T.);
#6994=EDGE_CURVE('',#5598,#5597,#4754,.T.);
#6995=EDGE_CURVE('',#5599,#5598,#4755,.T.);
#6996=EDGE_CURVE('',#5600,#5599,#4756,.T.);
#6997=EDGE_CURVE('',#5601,#5600,#4757,.T.);
#6998=EDGE_CURVE('',#5596,#5601,#4758,.T.);
#6999=EDGE_CURVE('',#5602,#5603,#4759,.T.);
#7000=EDGE_CURVE('',#5604,#5602,#3170,.T.);
#7001=EDGE_CURVE('',#5605,#5604,#4760,.T.);
#7002=EDGE_CURVE('',#5603,#5605,#3171,.T.);
#7003=EDGE_CURVE('',#5606,#5606,#4761,.T.);
#7004=EDGE_CURVE('',#5606,#5607,#3172,.T.);
#7005=EDGE_CURVE('',#5607,#5607,#4762,.T.);
#7006=EDGE_CURVE('',#5608,#5608,#4763,.T.);
#7007=EDGE_CURVE('',#5608,#5609,#3173,.T.);
#7008=EDGE_CURVE('',#5609,#5609,#4764,.T.);
#7009=EDGE_CURVE('',#5610,#5610,#4765,.T.);
#7010=EDGE_CURVE('',#5610,#5611,#3174,.T.);
#7011=EDGE_CURVE('',#5611,#5611,#4766,.T.);
#7012=EDGE_CURVE('',#5612,#5612,#4767,.T.);
#7013=EDGE_CURVE('',#5612,#5613,#3175,.T.);
#7014=EDGE_CURVE('',#5613,#5614,#4768,.T.);
#7015=EDGE_CURVE('',#5614,#5615,#4769,.T.);
#7016=EDGE_CURVE('',#5615,#5613,#4770,.T.);
#7017=EDGE_CURVE('',#5616,#5617,#782,.F.);
#7018=EDGE_CURVE('',#5617,#5614,#35,.T.);
#7019=EDGE_CURVE('',#5613,#5618,#3176,.T.);
#7020=EDGE_CURVE('',#5618,#5619,#4771,.T.);
#7021=EDGE_CURVE('',#5619,#5620,#4772,.T.);
#7022=EDGE_CURVE('',#5620,#5621,#4773,.T.);
#7023=EDGE_CURVE('',#5621,#5622,#4774,.T.);
#7024=EDGE_CURVE('',#5622,#5618,#4775,.T.);
#7025=EDGE_CURVE('',#5615,#5616,#879,.T.);
#7026=EDGE_CURVE('',#5570,#5623,#3177,.T.);
#7027=EDGE_CURVE('',#5623,#5624,#880,.T.);
#7028=EDGE_CURVE('',#5624,#5625,#881,.T.);
#7029=EDGE_CURVE('',#5625,#5626,#3178,.T.);
#7030=EDGE_CURVE('',#5626,#5627,#882,.T.);
#7031=EDGE_CURVE('',#5627,#5628,#883,.T.);
#7032=EDGE_CURVE('',#5628,#5569,#3179,.T.);
#7033=EDGE_CURVE('',#5628,#5629,#884,.T.);
#7034=EDGE_CURVE('',#5630,#5629,#885,.T.);
#7035=EDGE_CURVE('',#5630,#5631,#3180,.T.);
#7036=EDGE_CURVE('',#5632,#5631,#886,.T.);
#7037=EDGE_CURVE('',#5632,#5623,#887,.T.);
#7038=EDGE_CURVE('',#5633,#5634,#3181,.T.);
#7039=EDGE_CURVE('',#5634,#5635,#3182,.T.);
#7040=EDGE_CURVE('',#5635,#5636,#3183,.T.);
#7041=EDGE_CURVE('',#5636,#5633,#3184,.T.);
#7042=EDGE_CURVE('',#5637,#5638,#3185,.T.);
#7043=EDGE_CURVE('',#5638,#5626,#888,.T.);
#7044=EDGE_CURVE('',#5625,#5637,#889,.T.);
#7045=EDGE_CURVE('',#5639,#5640,#3186,.T.);
#7046=EDGE_CURVE('',#5640,#5638,#3187,.T.);
#7047=EDGE_CURVE('',#5637,#5639,#3188,.T.);
#7048=EDGE_CURVE('',#5622,#5640,#4776,.T.);
#7049=EDGE_CURVE('',#5639,#5619,#4777,.T.);
#7050=EDGE_CURVE('',#5633,#5621,#4778,.T.);
#7051=EDGE_CURVE('',#5620,#5634,#4779,.T.);
#7052=EDGE_CURVE('',#5641,#5642,#3189,.T.);
#7053=EDGE_CURVE('',#5643,#5641,#3190,.T.);
#7054=EDGE_CURVE('',#5644,#5643,#3191,.T.);
#7055=EDGE_CURVE('',#5645,#5644,#3192,.T.);
#7056=EDGE_CURVE('',#5646,#5645,#3193,.T.);
#7057=EDGE_CURVE('',#5642,#5646,#3194,.T.);
#7058=EDGE_CURVE('',#5647,#5642,#3195,.T.);
#7059=EDGE_CURVE('',#5647,#5648,#3196,.T.);
#7060=EDGE_CURVE('',#5648,#5641,#3197,.T.);
#7061=EDGE_CURVE('',#5649,#5646,#3198,.T.);
#7062=EDGE_CURVE('',#5649,#5647,#3199,.T.);
#7063=EDGE_CURVE('',#5650,#5645,#3200,.T.);
#7064=EDGE_CURVE('',#5650,#5649,#3201,.T.);
#7065=EDGE_CURVE('',#5651,#5644,#3202,.T.);
#7066=EDGE_CURVE('',#5651,#5650,#3203,.T.);
#7067=EDGE_CURVE('',#5652,#5643,#3204,.T.);
#7068=EDGE_CURVE('',#5652,#5651,#3205,.T.);
#7069=EDGE_CURVE('',#5648,#5652,#3206,.T.);
#7070=EDGE_CURVE('',#5653,#5654,#3207,.T.);
#7071=EDGE_CURVE('',#5654,#5655,#3208,.T.);
#7072=EDGE_CURVE('',#5655,#5656,#3209,.T.);
#7073=EDGE_CURVE('',#5656,#5657,#3210,.T.);
#7074=EDGE_CURVE('',#5657,#5658,#3211,.T.);
#7075=EDGE_CURVE('',#5658,#5653,#3212,.T.);
#7076=EDGE_CURVE('',#5659,#5660,#3213,.T.);
#7077=EDGE_CURVE('',#5661,#5659,#3214,.T.);
#7078=EDGE_CURVE('',#5662,#5661,#3215,.T.);
#7079=EDGE_CURVE('',#5662,#5663,#3216,.T.);
#7080=EDGE_CURVE('',#5663,#5604,#3217,.T.);
#7081=EDGE_CURVE('',#5602,#5664,#3218,.T.);
#7082=EDGE_CURVE('',#5664,#5660,#3219,.T.);
#7083=EDGE_CURVE('',#5614,#5663,#3220,.T.);
#7084=EDGE_CURVE('',#5665,#5662,#3221,.T.);
#7085=EDGE_CURVE('',#5666,#5665,#3222,.T.);
#7086=EDGE_CURVE('',#5666,#5660,#3223,.T.);
#7087=EDGE_CURVE('',#5615,#5664,#3224,.T.);
#7088=EDGE_CURVE('',#5616,#5603,#3225,.T.);
#7089=EDGE_CURVE('',#5617,#5605,#3226,.T.);
#7090=EDGE_CURVE('',#5667,#5661,#3227,.T.);
#7091=EDGE_CURVE('',#5667,#5668,#4780,.T.);
#7092=EDGE_CURVE('',#5665,#5668,#3228,.T.);
#7093=EDGE_CURVE('',#5669,#5659,#3229,.T.);
#7094=EDGE_CURVE('',#5669,#5667,#3230,.T.);
#7095=EDGE_CURVE('',#5670,#5666,#3231,.T.);
#7096=EDGE_CURVE('',#5670,#5669,#4781,.T.);
#7097=EDGE_CURVE('',#5668,#5670,#3232,.T.);
#7098=EDGE_CURVE('',#5596,#5671,#3233,.T.);
#7099=EDGE_CURVE('',#5671,#5601,#3234,.T.);
#7100=EDGE_CURVE('',#5601,#5672,#3235,.T.);
#7101=EDGE_CURVE('',#5672,#5600,#3236,.T.);
#7102=EDGE_CURVE('',#5600,#5673,#3237,.T.);
#7103=EDGE_CURVE('',#5673,#5599,#3238,.T.);
#7104=EDGE_CURVE('',#5599,#5674,#3239,.T.);
#7105=EDGE_CURVE('',#5674,#5598,#3240,.T.);
#7106=EDGE_CURVE('',#5598,#5675,#3241,.T.);
#7107=EDGE_CURVE('',#5675,#5597,#3242,.T.);
#7108=EDGE_CURVE('',#5597,#5676,#3243,.T.);
#7109=EDGE_CURVE('',#5676,#5596,#3244,.T.);
#7110=EDGE_CURVE('',#5584,#5677,#3245,.T.);
#7111=EDGE_CURVE('',#5677,#5678,#783,.T.);
#7112=EDGE_CURVE('',#5678,#5674,#3246,.T.);
#7113=EDGE_CURVE('',#5585,#5675,#3247,.T.);
#7114=EDGE_CURVE('',#5679,#5586,#3248,.T.);
#7115=EDGE_CURVE('',#5680,#5676,#3249,.T.);
#7116=EDGE_CURVE('',#5680,#5679,#784,.T.);
#7117=EDGE_CURVE('',#5681,#5682,#3250,.T.);
#7118=EDGE_CURVE('',#5682,#5680,#785,.T.);
#7119=EDGE_CURVE('',#5683,#5671,#3251,.T.);
#7120=EDGE_CURVE('',#5683,#5681,#786,.T.);
#7121=EDGE_CURVE('',#5589,#5684,#3252,.T.);
#7122=EDGE_CURVE('',#5684,#5683,#787,.T.);
#7123=EDGE_CURVE('',#5588,#5672,#3253,.T.);
#7124=EDGE_CURVE('',#5685,#5673,#3254,.T.);
#7125=EDGE_CURVE('',#5685,#5686,#788,.T.);
#7126=EDGE_CURVE('',#5686,#5590,#3255,.T.);
#7127=EDGE_CURVE('',#5678,#5687,#789,.T.);
#7128=EDGE_CURVE('',#5687,#5688,#3256,.T.);
#7129=EDGE_CURVE('',#5688,#5685,#790,.T.);
#7130=EDGE_CURVE('',#5592,#5689,#791,.T.);
#7131=EDGE_CURVE('',#5689,#5581,#792,.T.);
#7132=EDGE_CURVE('',#5582,#5690,#793,.T.);
#7133=EDGE_CURVE('',#5690,#5593,#794,.T.);
#7134=EDGE_CURVE('',#5583,#5677,#3257,.T.);
#7135=EDGE_CURVE('',#5679,#5587,#3258,.T.);
#7136=EDGE_CURVE('',#5687,#5691,#3259,.T.);
#7137=EDGE_CURVE('',#5691,#5688,#3260,.T.);
#7138=EDGE_CURVE('',#5681,#5692,#3261,.T.);
#7139=EDGE_CURVE('',#5692,#5682,#3262,.T.);
#7140=EDGE_CURVE('',#5686,#5591,#3263,.T.);
#7141=EDGE_CURVE('',#5594,#5684,#3264,.T.);
#7142=EDGE_CURVE('',#5692,#5690,#795,.T.);
#7143=EDGE_CURVE('',#5689,#5691,#796,.T.);
#7144=EDGE_CURVE('',#5693,#5694,#890,.T.);
#7145=EDGE_CURVE('',#5694,#5622,#3265,.T.);
#7146=EDGE_CURVE('',#5621,#5695,#3266,.T.);
#7147=EDGE_CURVE('',#5695,#5693,#891,.T.);
#7148=EDGE_CURVE('',#5619,#5696,#3267,.T.);
#7149=EDGE_CURVE('',#5696,#5697,#892,.T.);
#7150=EDGE_CURVE('',#5697,#5698,#893,.T.);
#7151=EDGE_CURVE('',#5698,#5620,#3268,.T.);
#7152=EDGE_CURVE('',#5696,#5637,#4782,.T.);
#7153=EDGE_CURVE('',#5697,#5625,#894,.T.);
#7154=EDGE_CURVE('',#5697,#5624,#4783,.T.);
#7155=EDGE_CURVE('',#5698,#5632,#4784,.T.);
#7156=EDGE_CURVE('',#5635,#5698,#895,.T.);
#7157=EDGE_CURVE('',#5635,#5631,#4785,.T.);
#7158=EDGE_CURVE('',#5638,#5694,#4786,.T.);
#7159=EDGE_CURVE('',#5636,#5630,#4787,.T.);
#7160=EDGE_CURVE('',#5695,#5636,#896,.T.);
#7161=EDGE_CURVE('',#5626,#5693,#897,.T.);
#7162=EDGE_CURVE('',#5695,#5629,#4788,.T.);
#7163=EDGE_CURVE('',#5627,#5693,#4789,.T.);
#7164=EDGE_CURVE('',#5649,#5657,#797,.T.);
#7165=EDGE_CURVE('',#5658,#5650,#798,.T.);
#7166=EDGE_CURVE('',#5653,#5651,#799,.T.);
#7167=EDGE_CURVE('',#5647,#5656,#800,.T.);
#7168=EDGE_CURVE('',#5654,#5652,#801,.T.);
#7169=EDGE_CURVE('',#5648,#5655,#802,.T.);
#9481=ORIENTED_EDGE('',*,*,#6953,.T.);
#9482=ORIENTED_EDGE('',*,*,#6954,.T.);
#9483=ORIENTED_EDGE('',*,*,#6955,.T.);
#9484=ORIENTED_EDGE('',*,*,#6954,.F.);
#9485=ORIENTED_EDGE('',*,*,#6956,.T.);
#9486=ORIENTED_EDGE('',*,*,#6957,.F.);
#9487=ORIENTED_EDGE('',*,*,#6958,.T.);
#9488=ORIENTED_EDGE('',*,*,#6959,.F.);
#9489=ORIENTED_EDGE('',*,*,#6960,.F.);
#9490=ORIENTED_EDGE('',*,*,#6958,.F.);
#9491=ORIENTED_EDGE('',*,*,#6961,.F.);
#9492=ORIENTED_EDGE('',*,*,#6962,.F.);
#9493=ORIENTED_EDGE('',*,*,#6963,.T.);
#9494=ORIENTED_EDGE('',*,*,#6964,.F.);
#9495=ORIENTED_EDGE('',*,*,#6963,.F.);
#9496=ORIENTED_EDGE('',*,*,#6965,.F.);
#9497=ORIENTED_EDGE('',*,*,#6966,.T.);
#9498=ORIENTED_EDGE('',*,*,#6967,.T.);
#9499=ORIENTED_EDGE('',*,*,#6966,.F.);
#9500=ORIENTED_EDGE('',*,*,#6968,.F.);
#9501=ORIENTED_EDGE('',*,*,#6969,.T.);
#9502=ORIENTED_EDGE('',*,*,#6970,.T.);
#9503=ORIENTED_EDGE('',*,*,#6969,.F.);
#9504=ORIENTED_EDGE('',*,*,#6953,.F.);
#9505=ORIENTED_EDGE('',*,*,#6956,.F.);
#9506=ORIENTED_EDGE('',*,*,#6971,.F.);
#9507=ORIENTED_EDGE('',*,*,#6972,.T.);
#9508=ORIENTED_EDGE('',*,*,#6973,.T.);
#9509=ORIENTED_EDGE('',*,*,#6972,.F.);
#9510=ORIENTED_EDGE('',*,*,#6974,.F.);
#9511=ORIENTED_EDGE('',*,*,#6975,.T.);
#9512=ORIENTED_EDGE('',*,*,#6976,.T.);
#9513=ORIENTED_EDGE('',*,*,#6975,.F.);
#9514=ORIENTED_EDGE('',*,*,#6977,.F.);
#9515=ORIENTED_EDGE('',*,*,#6978,.F.);
#9516=ORIENTED_EDGE('',*,*,#6979,.F.);
#9517=ORIENTED_EDGE('',*,*,#6980,.F.);
#9518=ORIENTED_EDGE('',*,*,#6981,.F.);
#9519=ORIENTED_EDGE('',*,*,#6982,.F.);
#9520=ORIENTED_EDGE('',*,*,#6983,.T.);
#9521=ORIENTED_EDGE('',*,*,#6984,.F.);
#9522=ORIENTED_EDGE('',*,*,#6985,.F.);
#9523=ORIENTED_EDGE('',*,*,#6986,.F.);
#9524=ORIENTED_EDGE('',*,*,#6987,.F.);
#9525=ORIENTED_EDGE('',*,*,#6988,.F.);
#9526=ORIENTED_EDGE('',*,*,#6989,.T.);
#9527=ORIENTED_EDGE('',*,*,#6990,.F.);
#9528=ORIENTED_EDGE('',*,*,#6991,.T.);
#9529=ORIENTED_EDGE('',*,*,#6992,.T.);
#9530=ORIENTED_EDGE('',*,*,#6993,.F.);
#9531=ORIENTED_EDGE('',*,*,#6994,.F.);
#9532=ORIENTED_EDGE('',*,*,#6995,.F.);
#9533=ORIENTED_EDGE('',*,*,#6996,.F.);
#9534=ORIENTED_EDGE('',*,*,#6997,.F.);
#9535=ORIENTED_EDGE('',*,*,#6998,.F.);
#9536=ORIENTED_EDGE('',*,*,#6992,.F.);
#9537=ORIENTED_EDGE('',*,*,#6999,.F.);
#9538=ORIENTED_EDGE('',*,*,#7000,.F.);
#9539=ORIENTED_EDGE('',*,*,#7001,.F.);
#9540=ORIENTED_EDGE('',*,*,#7002,.F.);
#9541=ORIENTED_EDGE('',*,*,#7003,.F.);
#9542=ORIENTED_EDGE('',*,*,#7004,.T.);
#9543=ORIENTED_EDGE('',*,*,#7005,.T.);
#9544=ORIENTED_EDGE('',*,*,#7004,.F.);
#9545=ORIENTED_EDGE('',*,*,#7006,.F.);
#9546=ORIENTED_EDGE('',*,*,#7007,.T.);
#9547=ORIENTED_EDGE('',*,*,#7008,.T.);
#9548=ORIENTED_EDGE('',*,*,#7007,.F.);
#9549=ORIENTED_EDGE('',*,*,#7009,.F.);
#9550=ORIENTED_EDGE('',*,*,#7010,.T.);
#9551=ORIENTED_EDGE('',*,*,#7011,.T.);
#9552=ORIENTED_EDGE('',*,*,#7010,.F.);
#9553=ORIENTED_EDGE('',*,*,#7012,.F.);
#9554=ORIENTED_EDGE('',*,*,#7013,.T.);
#9555=ORIENTED_EDGE('',*,*,#7014,.T.);
#9556=ORIENTED_EDGE('',*,*,#7015,.T.);
#9557=ORIENTED_EDGE('',*,*,#7016,.T.);
#9558=ORIENTED_EDGE('',*,*,#7013,.F.);
#9559=ORIENTED_EDGE('',*,*,#7017,.T.);
#9560=ORIENTED_EDGE('',*,*,#7018,.T.);
#9561=ORIENTED_EDGE('',*,*,#7014,.F.);
#9562=ORIENTED_EDGE('',*,*,#7019,.T.);
#9563=ORIENTED_EDGE('',*,*,#7020,.T.);
#9564=ORIENTED_EDGE('',*,*,#7021,.T.);
#9565=ORIENTED_EDGE('',*,*,#7022,.T.);
#9566=ORIENTED_EDGE('',*,*,#7023,.T.);
#9567=ORIENTED_EDGE('',*,*,#7024,.T.);
#9568=ORIENTED_EDGE('',*,*,#7019,.F.);
#9569=ORIENTED_EDGE('',*,*,#7016,.F.);
#9570=ORIENTED_EDGE('',*,*,#7025,.T.);
#9571=ORIENTED_EDGE('',*,*,#6961,.T.);
#9572=ORIENTED_EDGE('',*,*,#6962,.T.);
#9573=ORIENTED_EDGE('',*,*,#7026,.T.);
#9574=ORIENTED_EDGE('',*,*,#7027,.T.);
#9575=ORIENTED_EDGE('',*,*,#7028,.T.);
#9576=ORIENTED_EDGE('',*,*,#7029,.T.);
#9577=ORIENTED_EDGE('',*,*,#7030,.T.);
#9578=ORIENTED_EDGE('',*,*,#7031,.T.);
#9579=ORIENTED_EDGE('',*,*,#7032,.T.);
#9580=ORIENTED_EDGE('',*,*,#6959,.T.);
#9581=ORIENTED_EDGE('',*,*,#6960,.T.);
#9582=ORIENTED_EDGE('',*,*,#7032,.F.);
#9583=ORIENTED_EDGE('',*,*,#7033,.T.);
#9584=ORIENTED_EDGE('',*,*,#7034,.F.);
#9585=ORIENTED_EDGE('',*,*,#7035,.T.);
#9586=ORIENTED_EDGE('',*,*,#7036,.F.);
#9587=ORIENTED_EDGE('',*,*,#7037,.T.);
#9588=ORIENTED_EDGE('',*,*,#7026,.F.);
#9589=ORIENTED_EDGE('',*,*,#7038,.T.);
#9590=ORIENTED_EDGE('',*,*,#7039,.T.);
#9591=ORIENTED_EDGE('',*,*,#7040,.T.);
#9592=ORIENTED_EDGE('',*,*,#7041,.T.);
#9593=ORIENTED_EDGE('',*,*,#6991,.F.);
#9594=ORIENTED_EDGE('',*,*,#7042,.T.);
#9595=ORIENTED_EDGE('',*,*,#7043,.T.);
#9596=ORIENTED_EDGE('',*,*,#7029,.F.);
#9597=ORIENTED_EDGE('',*,*,#7044,.T.);
#9598=ORIENTED_EDGE('',*,*,#7045,.T.);
#9599=ORIENTED_EDGE('',*,*,#7046,.T.);
#9600=ORIENTED_EDGE('',*,*,#7042,.F.);
#9601=ORIENTED_EDGE('',*,*,#7047,.T.);
#9602=ORIENTED_EDGE('',*,*,#6957,.T.);
#9603=ORIENTED_EDGE('',*,*,#6976,.F.);
#9604=ORIENTED_EDGE('',*,*,#6964,.T.);
#9605=ORIENTED_EDGE('',*,*,#6974,.T.);
#9606=ORIENTED_EDGE('',*,*,#7024,.F.);
#9607=ORIENTED_EDGE('',*,*,#7048,.T.);
#9608=ORIENTED_EDGE('',*,*,#7045,.F.);
#9609=ORIENTED_EDGE('',*,*,#7049,.T.);
#9610=ORIENTED_EDGE('',*,*,#7020,.F.);
#9611=ORIENTED_EDGE('',*,*,#7038,.F.);
#9612=ORIENTED_EDGE('',*,*,#7050,.T.);
#9613=ORIENTED_EDGE('',*,*,#7022,.F.);
#9614=ORIENTED_EDGE('',*,*,#7051,.T.);
#9615=ORIENTED_EDGE('',*,*,#7012,.T.);
#9616=ORIENTED_EDGE('',*,*,#7011,.F.);
#9617=ORIENTED_EDGE('',*,*,#7009,.T.);
#9618=ORIENTED_EDGE('',*,*,#7008,.F.);
#9619=ORIENTED_EDGE('',*,*,#7006,.T.);
#9620=ORIENTED_EDGE('',*,*,#7005,.F.);
#9621=ORIENTED_EDGE('',*,*,#7003,.T.);
#9622=ORIENTED_EDGE('',*,*,#7052,.F.);
#9623=ORIENTED_EDGE('',*,*,#7053,.F.);
#9624=ORIENTED_EDGE('',*,*,#7054,.F.);
#9625=ORIENTED_EDGE('',*,*,#7055,.F.);
#9626=ORIENTED_EDGE('',*,*,#7056,.F.);
#9627=ORIENTED_EDGE('',*,*,#7057,.F.);
#9628=ORIENTED_EDGE('',*,*,#7058,.F.);
#9629=ORIENTED_EDGE('',*,*,#7059,.T.);
#9630=ORIENTED_EDGE('',*,*,#7060,.T.);
#9631=ORIENTED_EDGE('',*,*,#7052,.T.);
#9632=ORIENTED_EDGE('',*,*,#7061,.F.);
#9633=ORIENTED_EDGE('',*,*,#7062,.T.);
#9634=ORIENTED_EDGE('',*,*,#7058,.T.);
#9635=ORIENTED_EDGE('',*,*,#7057,.T.);
#9636=ORIENTED_EDGE('',*,*,#7063,.F.);
#9637=ORIENTED_EDGE('',*,*,#7064,.T.);
#9638=ORIENTED_EDGE('',*,*,#7061,.T.);
#9639=ORIENTED_EDGE('',*,*,#7056,.T.);
#9640=ORIENTED_EDGE('',*,*,#7065,.F.);
#9641=ORIENTED_EDGE('',*,*,#7066,.T.);
#9642=ORIENTED_EDGE('',*,*,#7063,.T.);
#9643=ORIENTED_EDGE('',*,*,#7055,.T.);
#9644=ORIENTED_EDGE('',*,*,#7067,.F.);
#9645=ORIENTED_EDGE('',*,*,#7068,.T.);
#9646=ORIENTED_EDGE('',*,*,#7065,.T.);
#9647=ORIENTED_EDGE('',*,*,#7054,.T.);
#9648=ORIENTED_EDGE('',*,*,#7060,.F.);
#9649=ORIENTED_EDGE('',*,*,#7069,.T.);
#9650=ORIENTED_EDGE('',*,*,#7067,.T.);
#9651=ORIENTED_EDGE('',*,*,#7053,.T.);
#9652=ORIENTED_EDGE('',*,*,#7070,.T.);
#9653=ORIENTED_EDGE('',*,*,#7071,.T.);
#9654=ORIENTED_EDGE('',*,*,#7072,.T.);
#9655=ORIENTED_EDGE('',*,*,#7073,.T.);
#9656=ORIENTED_EDGE('',*,*,#7074,.T.);
#9657=ORIENTED_EDGE('',*,*,#7075,.T.);
#9658=ORIENTED_EDGE('',*,*,#6967,.F.);
#9659=ORIENTED_EDGE('',*,*,#7076,.F.);
#9660=ORIENTED_EDGE('',*,*,#7077,.F.);
#9661=ORIENTED_EDGE('',*,*,#7078,.F.);
#9662=ORIENTED_EDGE('',*,*,#7079,.T.);
#9663=ORIENTED_EDGE('',*,*,#7080,.T.);
#9664=ORIENTED_EDGE('',*,*,#7000,.T.);
#9665=ORIENTED_EDGE('',*,*,#7081,.T.);
#9666=ORIENTED_EDGE('',*,*,#7082,.T.);
#9667=ORIENTED_EDGE('',*,*,#7015,.F.);
#9668=ORIENTED_EDGE('',*,*,#7083,.T.);
#9669=ORIENTED_EDGE('',*,*,#7079,.F.);
#9670=ORIENTED_EDGE('',*,*,#7084,.F.);
#9671=ORIENTED_EDGE('',*,*,#7085,.F.);
#9672=ORIENTED_EDGE('',*,*,#7086,.T.);
#9673=ORIENTED_EDGE('',*,*,#7082,.F.);
#9674=ORIENTED_EDGE('',*,*,#7087,.F.);
#9675=ORIENTED_EDGE('',*,*,#7081,.F.);
#9676=ORIENTED_EDGE('',*,*,#6999,.T.);
#9677=ORIENTED_EDGE('',*,*,#7088,.F.);
#9678=ORIENTED_EDGE('',*,*,#7025,.F.);
#9679=ORIENTED_EDGE('',*,*,#7087,.T.);
#9680=ORIENTED_EDGE('',*,*,#6973,.F.);
#9681=ORIENTED_EDGE('',*,*,#7089,.T.);
#9682=ORIENTED_EDGE('',*,*,#7001,.T.);
#9683=ORIENTED_EDGE('',*,*,#7080,.F.);
#9684=ORIENTED_EDGE('',*,*,#7083,.F.);
#9685=ORIENTED_EDGE('',*,*,#7018,.F.);
#9686=ORIENTED_EDGE('',*,*,#6971,.T.);
#9687=ORIENTED_EDGE('',*,*,#7088,.T.);
#9688=ORIENTED_EDGE('',*,*,#7002,.T.);
#9689=ORIENTED_EDGE('',*,*,#7089,.F.);
#9690=ORIENTED_EDGE('',*,*,#7017,.F.);
#9691=ORIENTED_EDGE('',*,*,#7090,.F.);
#9692=ORIENTED_EDGE('',*,*,#7091,.T.);
#9693=ORIENTED_EDGE('',*,*,#7092,.F.);
#9694=ORIENTED_EDGE('',*,*,#7084,.T.);
#9695=ORIENTED_EDGE('',*,*,#7078,.T.);
#9696=ORIENTED_EDGE('',*,*,#7093,.F.);
#9697=ORIENTED_EDGE('',*,*,#7094,.T.);
#9698=ORIENTED_EDGE('',*,*,#7090,.T.);
#9699=ORIENTED_EDGE('',*,*,#7077,.T.);
#9700=ORIENTED_EDGE('',*,*,#7095,.F.);
#9701=ORIENTED_EDGE('',*,*,#7096,.T.);
#9702=ORIENTED_EDGE('',*,*,#7093,.T.);
#9703=ORIENTED_EDGE('',*,*,#7076,.T.);
#9704=ORIENTED_EDGE('',*,*,#7086,.F.);
#9705=ORIENTED_EDGE('',*,*,#7092,.T.);
#9706=ORIENTED_EDGE('',*,*,#7097,.T.);
#9707=ORIENTED_EDGE('',*,*,#7095,.T.);
#9708=ORIENTED_EDGE('',*,*,#7085,.T.);
#9709=ORIENTED_EDGE('',*,*,#7098,.F.);
#9710=ORIENTED_EDGE('',*,*,#6998,.T.);
#9711=ORIENTED_EDGE('',*,*,#7099,.F.);
#9712=ORIENTED_EDGE('',*,*,#7100,.F.);
#9713=ORIENTED_EDGE('',*,*,#6997,.T.);
#9714=ORIENTED_EDGE('',*,*,#7101,.F.);
#9715=ORIENTED_EDGE('',*,*,#7102,.F.);
#9716=ORIENTED_EDGE('',*,*,#6996,.T.);
#9717=ORIENTED_EDGE('',*,*,#7103,.F.);
#9718=ORIENTED_EDGE('',*,*,#7104,.F.);
#9719=ORIENTED_EDGE('',*,*,#6995,.T.);
#9720=ORIENTED_EDGE('',*,*,#7105,.F.);
#9721=ORIENTED_EDGE('',*,*,#7106,.F.);
#9722=ORIENTED_EDGE('',*,*,#6994,.T.);
#9723=ORIENTED_EDGE('',*,*,#7107,.F.);
#9724=ORIENTED_EDGE('',*,*,#7108,.F.);
#9725=ORIENTED_EDGE('',*,*,#6993,.T.);
#9726=ORIENTED_EDGE('',*,*,#7109,.F.);
#9727=ORIENTED_EDGE('',*,*,#7110,.T.);
#9728=ORIENTED_EDGE('',*,*,#7111,.T.);
#9729=ORIENTED_EDGE('',*,*,#7112,.T.);
#9730=ORIENTED_EDGE('',*,*,#7105,.T.);
#9731=ORIENTED_EDGE('',*,*,#7106,.T.);
#9732=ORIENTED_EDGE('',*,*,#7113,.F.);
#9733=ORIENTED_EDGE('',*,*,#6980,.T.);
#9734=ORIENTED_EDGE('',*,*,#7114,.T.);
#9735=ORIENTED_EDGE('',*,*,#6981,.T.);
#9736=ORIENTED_EDGE('',*,*,#7113,.T.);
#9737=ORIENTED_EDGE('',*,*,#7107,.T.);
#9738=ORIENTED_EDGE('',*,*,#7108,.T.);
#9739=ORIENTED_EDGE('',*,*,#7115,.F.);
#9740=ORIENTED_EDGE('',*,*,#7116,.T.);
#9741=ORIENTED_EDGE('',*,*,#7117,.T.);
#9742=ORIENTED_EDGE('',*,*,#7118,.T.);
#9743=ORIENTED_EDGE('',*,*,#7115,.T.);
#9744=ORIENTED_EDGE('',*,*,#7109,.T.);
#9745=ORIENTED_EDGE('',*,*,#7098,.T.);
#9746=ORIENTED_EDGE('',*,*,#7119,.F.);
#9747=ORIENTED_EDGE('',*,*,#7120,.T.);
#9748=ORIENTED_EDGE('',*,*,#7121,.T.);
#9749=ORIENTED_EDGE('',*,*,#7122,.T.);
#9750=ORIENTED_EDGE('',*,*,#7119,.T.);
#9751=ORIENTED_EDGE('',*,*,#7099,.T.);
#9752=ORIENTED_EDGE('',*,*,#7100,.T.);
#9753=ORIENTED_EDGE('',*,*,#7123,.F.);
#9754=ORIENTED_EDGE('',*,*,#6984,.T.);
#9755=ORIENTED_EDGE('',*,*,#7124,.F.);
#9756=ORIENTED_EDGE('',*,*,#7125,.T.);
#9757=ORIENTED_EDGE('',*,*,#7126,.T.);
#9758=ORIENTED_EDGE('',*,*,#6985,.T.);
#9759=ORIENTED_EDGE('',*,*,#7123,.T.);
#9760=ORIENTED_EDGE('',*,*,#7101,.T.);
#9761=ORIENTED_EDGE('',*,*,#7102,.T.);
#9762=ORIENTED_EDGE('',*,*,#7112,.F.);
#9763=ORIENTED_EDGE('',*,*,#7127,.T.);
#9764=ORIENTED_EDGE('',*,*,#7128,.T.);
#9765=ORIENTED_EDGE('',*,*,#7129,.T.);
#9766=ORIENTED_EDGE('',*,*,#7124,.T.);
#9767=ORIENTED_EDGE('',*,*,#7103,.T.);
#9768=ORIENTED_EDGE('',*,*,#7104,.T.);
#9769=ORIENTED_EDGE('',*,*,#7130,.T.);
#9770=ORIENTED_EDGE('',*,*,#7131,.T.);
#9771=ORIENTED_EDGE('',*,*,#6977,.T.);
#9772=ORIENTED_EDGE('',*,*,#7132,.T.);
#9773=ORIENTED_EDGE('',*,*,#7133,.T.);
#9774=ORIENTED_EDGE('',*,*,#6988,.T.);
#9775=ORIENTED_EDGE('',*,*,#6970,.F.);
#9776=ORIENTED_EDGE('',*,*,#6979,.T.);
#9777=ORIENTED_EDGE('',*,*,#7134,.T.);
#9778=ORIENTED_EDGE('',*,*,#7110,.F.);
#9779=ORIENTED_EDGE('',*,*,#7135,.T.);
#9780=ORIENTED_EDGE('',*,*,#6982,.T.);
#9781=ORIENTED_EDGE('',*,*,#7114,.F.);
#9782=ORIENTED_EDGE('',*,*,#7128,.F.);
#9783=ORIENTED_EDGE('',*,*,#7136,.T.);
#9784=ORIENTED_EDGE('',*,*,#7137,.T.);
#9785=ORIENTED_EDGE('',*,*,#7138,.T.);
#9786=ORIENTED_EDGE('',*,*,#7139,.T.);
#9787=ORIENTED_EDGE('',*,*,#7117,.F.);
#9788=ORIENTED_EDGE('',*,*,#7126,.F.);
#9789=ORIENTED_EDGE('',*,*,#7140,.T.);
#9790=ORIENTED_EDGE('',*,*,#6986,.T.);
#9791=ORIENTED_EDGE('',*,*,#6990,.T.);
#9792=ORIENTED_EDGE('',*,*,#7141,.T.);
#9793=ORIENTED_EDGE('',*,*,#7121,.F.);
#9794=ORIENTED_EDGE('',*,*,#6989,.F.);
#9795=ORIENTED_EDGE('',*,*,#7133,.F.);
#9796=ORIENTED_EDGE('',*,*,#7142,.F.);
#9797=ORIENTED_EDGE('',*,*,#7138,.F.);
#9798=ORIENTED_EDGE('',*,*,#7120,.F.);
#9799=ORIENTED_EDGE('',*,*,#7122,.F.);
#9800=ORIENTED_EDGE('',*,*,#7141,.F.);
#9801=ORIENTED_EDGE('',*,*,#7142,.T.);
#9802=ORIENTED_EDGE('',*,*,#7132,.F.);
#9803=ORIENTED_EDGE('',*,*,#6983,.F.);
#9804=ORIENTED_EDGE('',*,*,#7135,.F.);
#9805=ORIENTED_EDGE('',*,*,#7116,.F.);
#9806=ORIENTED_EDGE('',*,*,#7118,.F.);
#9807=ORIENTED_EDGE('',*,*,#7139,.F.);
#9808=ORIENTED_EDGE('',*,*,#7129,.F.);
#9809=ORIENTED_EDGE('',*,*,#7137,.F.);
#9810=ORIENTED_EDGE('',*,*,#7143,.F.);
#9811=ORIENTED_EDGE('',*,*,#7130,.F.);
#9812=ORIENTED_EDGE('',*,*,#6987,.T.);
#9813=ORIENTED_EDGE('',*,*,#7140,.F.);
#9814=ORIENTED_EDGE('',*,*,#7125,.F.);
#9815=ORIENTED_EDGE('',*,*,#7134,.F.);
#9816=ORIENTED_EDGE('',*,*,#6978,.T.);
#9817=ORIENTED_EDGE('',*,*,#7131,.F.);
#9818=ORIENTED_EDGE('',*,*,#7143,.T.);
#9819=ORIENTED_EDGE('',*,*,#7136,.F.);
#9820=ORIENTED_EDGE('',*,*,#7127,.F.);
#9821=ORIENTED_EDGE('',*,*,#7111,.F.);
#9822=ORIENTED_EDGE('',*,*,#7144,.T.);
#9823=ORIENTED_EDGE('',*,*,#7145,.T.);
#9824=ORIENTED_EDGE('',*,*,#7023,.F.);
#9825=ORIENTED_EDGE('',*,*,#7146,.T.);
#9826=ORIENTED_EDGE('',*,*,#7147,.T.);
#9827=ORIENTED_EDGE('',*,*,#7021,.F.);
#9828=ORIENTED_EDGE('',*,*,#7148,.T.);
#9829=ORIENTED_EDGE('',*,*,#7149,.T.);
#9830=ORIENTED_EDGE('',*,*,#7150,.T.);
#9831=ORIENTED_EDGE('',*,*,#7151,.T.);
#9832=ORIENTED_EDGE('',*,*,#6968,.T.);
#9833=ORIENTED_EDGE('',*,*,#6965,.T.);
#9834=ORIENTED_EDGE('',*,*,#6955,.F.);
#9835=ORIENTED_EDGE('',*,*,#7049,.F.);
#9836=ORIENTED_EDGE('',*,*,#7047,.F.);
#9837=ORIENTED_EDGE('',*,*,#7152,.F.);
#9838=ORIENTED_EDGE('',*,*,#7148,.F.);
#9839=ORIENTED_EDGE('',*,*,#7152,.T.);
#9840=ORIENTED_EDGE('',*,*,#7044,.F.);
#9841=ORIENTED_EDGE('',*,*,#7153,.F.);
#9842=ORIENTED_EDGE('',*,*,#7149,.F.);
#9843=ORIENTED_EDGE('',*,*,#7153,.T.);
#9844=ORIENTED_EDGE('',*,*,#7028,.F.);
#9845=ORIENTED_EDGE('',*,*,#7154,.F.);
#9846=ORIENTED_EDGE('',*,*,#7154,.T.);
#9847=ORIENTED_EDGE('',*,*,#7027,.F.);
#9848=ORIENTED_EDGE('',*,*,#7037,.F.);
#9849=ORIENTED_EDGE('',*,*,#7155,.F.);
#9850=ORIENTED_EDGE('',*,*,#7150,.F.);
#9851=ORIENTED_EDGE('',*,*,#7051,.F.);
#9852=ORIENTED_EDGE('',*,*,#7151,.F.);
#9853=ORIENTED_EDGE('',*,*,#7156,.F.);
#9854=ORIENTED_EDGE('',*,*,#7039,.F.);
#9855=ORIENTED_EDGE('',*,*,#7155,.T.);
#9856=ORIENTED_EDGE('',*,*,#7036,.T.);
#9857=ORIENTED_EDGE('',*,*,#7157,.F.);
#9858=ORIENTED_EDGE('',*,*,#7156,.T.);
#9859=ORIENTED_EDGE('',*,*,#7048,.F.);
#9860=ORIENTED_EDGE('',*,*,#7145,.F.);
#9861=ORIENTED_EDGE('',*,*,#7158,.F.);
#9862=ORIENTED_EDGE('',*,*,#7046,.F.);
#9863=ORIENTED_EDGE('',*,*,#7157,.T.);
#9864=ORIENTED_EDGE('',*,*,#7035,.F.);
#9865=ORIENTED_EDGE('',*,*,#7159,.F.);
#9866=ORIENTED_EDGE('',*,*,#7040,.F.);
#9867=ORIENTED_EDGE('',*,*,#7050,.F.);
#9868=ORIENTED_EDGE('',*,*,#7041,.F.);
#9869=ORIENTED_EDGE('',*,*,#7160,.F.);
#9870=ORIENTED_EDGE('',*,*,#7146,.F.);
#9871=ORIENTED_EDGE('',*,*,#7158,.T.);
#9872=ORIENTED_EDGE('',*,*,#7144,.F.);
#9873=ORIENTED_EDGE('',*,*,#7161,.F.);
#9874=ORIENTED_EDGE('',*,*,#7043,.F.);
#9875=ORIENTED_EDGE('',*,*,#7159,.T.);
#9876=ORIENTED_EDGE('',*,*,#7034,.T.);
#9877=ORIENTED_EDGE('',*,*,#7162,.F.);
#9878=ORIENTED_EDGE('',*,*,#7160,.T.);
#9879=ORIENTED_EDGE('',*,*,#7030,.F.);
#9880=ORIENTED_EDGE('',*,*,#7161,.T.);
#9881=ORIENTED_EDGE('',*,*,#7163,.F.);
#9882=ORIENTED_EDGE('',*,*,#7162,.T.);
#9883=ORIENTED_EDGE('',*,*,#7033,.F.);
#9884=ORIENTED_EDGE('',*,*,#7031,.F.);
#9885=ORIENTED_EDGE('',*,*,#7163,.T.);
#9886=ORIENTED_EDGE('',*,*,#7147,.F.);
#9887=ORIENTED_EDGE('',*,*,#7164,.F.);
#9888=ORIENTED_EDGE('',*,*,#7064,.F.);
#9889=ORIENTED_EDGE('',*,*,#7165,.F.);
#9890=ORIENTED_EDGE('',*,*,#7074,.F.);
#9891=ORIENTED_EDGE('',*,*,#7165,.T.);
#9892=ORIENTED_EDGE('',*,*,#7066,.F.);
#9893=ORIENTED_EDGE('',*,*,#7166,.F.);
#9894=ORIENTED_EDGE('',*,*,#7075,.F.);
#9895=ORIENTED_EDGE('',*,*,#7164,.T.);
#9896=ORIENTED_EDGE('',*,*,#7073,.F.);
#9897=ORIENTED_EDGE('',*,*,#7167,.F.);
#9898=ORIENTED_EDGE('',*,*,#7062,.F.);
#9899=ORIENTED_EDGE('',*,*,#7166,.T.);
#9900=ORIENTED_EDGE('',*,*,#7068,.F.);
#9901=ORIENTED_EDGE('',*,*,#7168,.F.);
#9902=ORIENTED_EDGE('',*,*,#7070,.F.);
#9903=ORIENTED_EDGE('',*,*,#7167,.T.);
#9904=ORIENTED_EDGE('',*,*,#7072,.F.);
#9905=ORIENTED_EDGE('',*,*,#7169,.F.);
#9906=ORIENTED_EDGE('',*,*,#7059,.F.);
#9907=ORIENTED_EDGE('',*,*,#7168,.T.);
#9908=ORIENTED_EDGE('',*,*,#7069,.F.);
#9909=ORIENTED_EDGE('',*,*,#7169,.T.);
#9910=ORIENTED_EDGE('',*,*,#7071,.F.);
#9911=ORIENTED_EDGE('',*,*,#7091,.F.);
#9912=ORIENTED_EDGE('',*,*,#7094,.F.);
#9913=ORIENTED_EDGE('',*,*,#7096,.F.);
#9914=ORIENTED_EDGE('',*,*,#7097,.F.);
#11305=CONICAL_SURFACE('',#13056,27.,0.158655262186402);
#11645=ADVANCED_FACE('',(#1563),#1099,.F.);
#11646=ADVANCED_FACE('',(#1564),#829,.T.);
#11647=ADVANCED_FACE('',(#1565),#830,.T.);
#11648=ADVANCED_FACE('',(#1566),#1100,.F.);
#11649=ADVANCED_FACE('',(#1567,#397),#1101,.F.);
#11650=ADVANCED_FACE('',(#1568),#1102,.F.);
#11651=ADVANCED_FACE('',(#1569),#1103,.F.);
#11652=ADVANCED_FACE('',(#1570),#1104,.T.);
#11653=ADVANCED_FACE('',(#1571),#1105,.T.);
#11654=ADVANCED_FACE('',(#1572),#1106,.T.);
#11655=ADVANCED_FACE('',(#1573),#1107,.T.);
#11656=ADVANCED_FACE('',(#1574),#1108,.T.);
#11657=ADVANCED_FACE('',(#1575),#1109,.T.);
#11658=ADVANCED_FACE('',(#1576),#1110,.T.);
#11659=ADVANCED_FACE('',(#1577),#1111,.T.);
#11660=ADVANCED_FACE('',(#1578),#11305,.T.);
#11661=ADVANCED_FACE('',(#1579),#1112,.T.);
#11662=ADVANCED_FACE('',(#1580,#398),#588,.F.);
#11663=ADVANCED_FACE('',(#1581),#1113,.F.);
#11664=ADVANCED_FACE('',(#1582),#589,.F.);
#11665=ADVANCED_FACE('',(#1583,#399),#590,.T.);
#11666=ADVANCED_FACE('',(#1584,#400),#591,.F.);
#11667=ADVANCED_FACE('',(#1585),#592,.T.);
#11668=ADVANCED_FACE('',(#1586),#593,.T.);
#11669=ADVANCED_FACE('',(#1587,#401),#594,.T.);
#11670=ADVANCED_FACE('',(#1588,#402),#595,.T.);
#11671=ADVANCED_FACE('',(#1589,#403),#596,.T.);
#11672=ADVANCED_FACE('',(#1590,#404),#597,.T.);
#11673=ADVANCED_FACE('',(#1591),#598,.F.);
#11674=ADVANCED_FACE('',(#1592),#599,.F.);
#11675=ADVANCED_FACE('',(#1593),#600,.F.);
#11676=ADVANCED_FACE('',(#1594),#601,.F.);
#11677=ADVANCED_FACE('',(#1595),#602,.F.);
#11678=ADVANCED_FACE('',(#1596),#603,.F.);
#11679=ADVANCED_FACE('',(#1597,#405),#604,.T.);
#11680=ADVANCED_FACE('',(#1598),#605,.T.);
#11681=ADVANCED_FACE('',(#1599),#606,.F.);
#11682=ADVANCED_FACE('',(#1600,#406),#607,.F.);
#11683=ADVANCED_FACE('',(#1601,#407),#608,.F.);
#11684=ADVANCED_FACE('',(#1602),#609,.F.);
#11685=ADVANCED_FACE('',(#1603),#610,.F.);
#11686=ADVANCED_FACE('',(#1604),#611,.F.);
#11687=ADVANCED_FACE('',(#1605),#612,.F.);
#11688=ADVANCED_FACE('',(#1606),#613,.F.);
#11689=ADVANCED_FACE('',(#1607),#614,.F.);
#11690=ADVANCED_FACE('',(#1608),#615,.F.);
#11691=ADVANCED_FACE('',(#1609),#616,.F.);
#11692=ADVANCED_FACE('',(#1610),#617,.F.);
#11693=ADVANCED_FACE('',(#1611),#618,.F.);
#11694=ADVANCED_FACE('',(#1612),#619,.F.);
#11695=ADVANCED_FACE('',(#1613),#620,.F.);
#11696=ADVANCED_FACE('',(#1614),#621,.F.);
#11697=ADVANCED_FACE('',(#1615),#622,.F.);
#11698=ADVANCED_FACE('',(#1616),#623,.F.);
#11699=ADVANCED_FACE('',(#1617),#624,.F.);
#11700=ADVANCED_FACE('',(#1618),#625,.F.);
#11701=ADVANCED_FACE('',(#1619,#408),#626,.T.);
#11702=ADVANCED_FACE('',(#1620),#627,.T.);
#11703=ADVANCED_FACE('',(#1621),#628,.T.);
#11704=ADVANCED_FACE('',(#1622),#629,.T.);
#11705=ADVANCED_FACE('',(#1623),#630,.T.);
#11706=ADVANCED_FACE('',(#1624),#631,.T.);
#11707=ADVANCED_FACE('',(#1625),#632,.T.);
#11708=ADVANCED_FACE('',(#1626),#1114,.T.);
#11709=ADVANCED_FACE('',(#1627),#1115,.T.);
#11710=ADVANCED_FACE('',(#1628),#1116,.T.);
#11711=ADVANCED_FACE('',(#1629),#1117,.T.);
#11712=ADVANCED_FACE('',(#1630),#1118,.T.);
#11713=ADVANCED_FACE('',(#1631),#1119,.T.);
#11714=ADVANCED_FACE('',(#1632),#633,.T.);
#11715=ADVANCED_FACE('',(#1633,#409),#634,.T.);
#11716=ADVANCED_FACE('',(#1634),#1120,.T.);
#11717=ADVANCED_FACE('',(#1635),#310,.T.);
#11718=ADVANCED_FACE('',(#1636),#311,.F.);
#11719=ADVANCED_FACE('',(#1637),#312,.F.);
#11720=ADVANCED_FACE('',(#1638),#1121,.T.);
#11721=ADVANCED_FACE('',(#1639),#313,.F.);
#11722=ADVANCED_FACE('',(#1640),#1122,.T.);
#11723=ADVANCED_FACE('',(#1641),#1123,.F.);
#11724=ADVANCED_FACE('',(#1642),#1124,.T.);
#11725=ADVANCED_FACE('',(#1643),#314,.T.);
#11726=ADVANCED_FACE('',(#1644),#315,.F.);
#11727=ADVANCED_FACE('',(#1645),#316,.F.);
#11728=ADVANCED_FACE('',(#1646),#317,.F.);
#11729=ADVANCED_FACE('',(#1647),#1125,.T.);
#11730=ADVANCED_FACE('',(#1648),#1126,.T.);
#11731=ADVANCED_FACE('',(#1649),#1127,.T.);
#11732=ADVANCED_FACE('',(#1650),#1128,.T.);
#11733=ADVANCED_FACE('',(#1651),#1129,.T.);
#11734=ADVANCED_FACE('',(#1652),#1130,.T.);
#11735=ADVANCED_FACE('',(#1653),#1131,.T.);
#12035=CLOSED_SHELL('',(#11645,#11646,#11647,#11648,#11649,#11650,#11651,
#11652,#11653,#11654,#11655,#11656,#11657,#11658,#11659,#11660,#11661,#11662,
#11663,#11664,#11665,#11666,#11667,#11668,#11669,#11670,#11671,#11672,#11673,
#11674,#11675,#11676,#11677,#11678,#11679,#11680,#11681,#11682,#11683,#11684,
#11685,#11686,#11687,#11688,#11689,#11690,#11691,#11692,#11693,#11694,#11695,
#11696,#11697,#11698,#11699,#11700,#11701,#11702,#11703,#11704,#11705,#11706,
#11707,#11708,#11709,#11710,#11711,#11712,#11713,#11714,#11715,#11716,#11717,
#11718,#11719,#11720,#11721,#11722,#11723,#11724,#11725,#11726,#11727,#11728,
#11729,#11730,#11731,#11732,#11733,#11734,#11735));
#12994=AXIS2_PLACEMENT_3D('',#19399,#15530,#15531);
#12995=AXIS2_PLACEMENT_3D('',#19400,#15532,#15533);
#12996=AXIS2_PLACEMENT_3D('',#19423,#15535,#15536);
#12997=AXIS2_PLACEMENT_3D('',#19442,#15537,#15538);
#12998=AXIS2_PLACEMENT_3D('',#19444,#15539,#15540);
#12999=AXIS2_PLACEMENT_3D('',#19446,#15541,#15542);
#13000=AXIS2_PLACEMENT_3D('',#19448,#15543,#15544);
#13001=AXIS2_PLACEMENT_3D('',#19449,#15545,#15546);
#13002=AXIS2_PLACEMENT_3D('',#19450,#15547,#15548);
#13003=AXIS2_PLACEMENT_3D('',#19453,#15549,#15550);
#13004=AXIS2_PLACEMENT_3D('',#19454,#15551,#15552);
#13005=AXIS2_PLACEMENT_3D('',#19456,#15553,#15554);
#13006=AXIS2_PLACEMENT_3D('',#19457,#15555,#15556);
#13007=AXIS2_PLACEMENT_3D('',#19458,#15557,#15558);
#13008=AXIS2_PLACEMENT_3D('',#19460,#15559,#15560);
#13009=AXIS2_PLACEMENT_3D('',#19463,#15562,#15563);
#13010=AXIS2_PLACEMENT_3D('',#19464,#15564,#15565);
#13011=AXIS2_PLACEMENT_3D('',#19466,#15566,#15567);
#13012=AXIS2_PLACEMENT_3D('',#19469,#15569,#15570);
#13013=AXIS2_PLACEMENT_3D('',#19470,#15571,#15572);
#13014=AXIS2_PLACEMENT_3D('',#19472,#15573,#15574);
#13015=AXIS2_PLACEMENT_3D('',#19475,#15576,#15577);
#13016=AXIS2_PLACEMENT_3D('',#19476,#15578,#15579);
#13017=AXIS2_PLACEMENT_3D('',#19478,#15580,#15581);
#13018=AXIS2_PLACEMENT_3D('',#19481,#15583,#15584);
#13019=AXIS2_PLACEMENT_3D('',#19482,#15585,#15586);
#13020=AXIS2_PLACEMENT_3D('',#19485,#15587,#15588);
#13021=AXIS2_PLACEMENT_3D('',#19487,#15589,#15590);
#13022=AXIS2_PLACEMENT_3D('',#19491,#15592,#15593);
#13023=AXIS2_PLACEMENT_3D('',#19493,#15594,#15595);
#13024=AXIS2_PLACEMENT_3D('',#19496,#15597,#15598);
#13025=AXIS2_PLACEMENT_3D('',#19497,#15599,#15600);
#13026=AXIS2_PLACEMENT_3D('',#19500,#15601,#15602);
#13027=AXIS2_PLACEMENT_3D('',#19502,#15603,#15604);
#13028=AXIS2_PLACEMENT_3D('',#19506,#15606,#15607);
#13029=AXIS2_PLACEMENT_3D('',#19508,#15608,#15609);
#13030=AXIS2_PLACEMENT_3D('',#19510,#15610,#15611);
#13031=AXIS2_PLACEMENT_3D('',#19512,#15613,#15614);
#13032=AXIS2_PLACEMENT_3D('',#19514,#15615,#15616);
#13033=AXIS2_PLACEMENT_3D('',#19518,#15618,#15619);
#13034=AXIS2_PLACEMENT_3D('',#19520,#15620,#15621);
#13035=AXIS2_PLACEMENT_3D('',#19522,#15622,#15623);
#13036=AXIS2_PLACEMENT_3D('',#19524,#15624,#15625);
#13037=AXIS2_PLACEMENT_3D('',#19526,#15626,#15627);
#13038=AXIS2_PLACEMENT_3D('',#19527,#15628,#15629);
#13039=AXIS2_PLACEMENT_3D('',#19528,#15630,#15631);
#13040=AXIS2_PLACEMENT_3D('',#19531,#15632,#15633);
#13041=AXIS2_PLACEMENT_3D('',#19535,#15635,#15636);
#13042=AXIS2_PLACEMENT_3D('',#19537,#15638,#15639);
#13043=AXIS2_PLACEMENT_3D('',#19539,#15640,#15641);
#13044=AXIS2_PLACEMENT_3D('',#19542,#15643,#15644);
#13045=AXIS2_PLACEMENT_3D('',#19543,#15645,#15646);
#13046=AXIS2_PLACEMENT_3D('',#19545,#15647,#15648);
#13047=AXIS2_PLACEMENT_3D('',#19548,#15650,#15651);
#13048=AXIS2_PLACEMENT_3D('',#19549,#15652,#15653);
#13049=AXIS2_PLACEMENT_3D('',#19551,#15654,#15655);
#13050=AXIS2_PLACEMENT_3D('',#19554,#15657,#15658);
#13051=AXIS2_PLACEMENT_3D('',#19555,#15659,#15660);
#13052=AXIS2_PLACEMENT_3D('',#19557,#15661,#15662);
#13053=AXIS2_PLACEMENT_3D('',#19561,#15664,#15665);
#13054=AXIS2_PLACEMENT_3D('',#19563,#15666,#15667);
#13055=AXIS2_PLACEMENT_3D('',#19564,#15668,#15669);
#13056=AXIS2_PLACEMENT_3D('',#19565,#15670,#15671);
#13057=AXIS2_PLACEMENT_3D('',#19568,#15672,#15673);
#13058=AXIS2_PLACEMENT_3D('',#19575,#15675,#15676);
#13059=AXIS2_PLACEMENT_3D('',#19577,#15677,#15678);
#13060=AXIS2_PLACEMENT_3D('',#19579,#15679,#15680);
#13061=AXIS2_PLACEMENT_3D('',#19581,#15681,#15682);
#13062=AXIS2_PLACEMENT_3D('',#19582,#15683,#15684);
#13063=AXIS2_PLACEMENT_3D('',#19587,#15685,#15686);
#13064=AXIS2_PLACEMENT_3D('',#19932,#15691,#15692);
#13065=AXIS2_PLACEMENT_3D('',#19941,#15697,#15698);
#13066=AXIS2_PLACEMENT_3D('',#20037,#15700,#15701);
#13067=AXIS2_PLACEMENT_3D('',#20043,#15705,#15706);
#13068=AXIS2_PLACEMENT_3D('',#20044,#15707,#15708);
#13069=AXIS2_PLACEMENT_3D('',#20045,#15709,#15710);
#13070=AXIS2_PLACEMENT_3D('',#20046,#15711,#15712);
#13071=AXIS2_PLACEMENT_3D('',#20047,#15713,#15714);
#13072=AXIS2_PLACEMENT_3D('',#20048,#15715,#15716);
#13073=AXIS2_PLACEMENT_3D('',#20049,#15717,#15718);
#13074=AXIS2_PLACEMENT_3D('',#20050,#15719,#15720);
#13075=AXIS2_PLACEMENT_3D('',#20051,#15721,#15722);
#13076=AXIS2_PLACEMENT_3D('',#20052,#15723,#15724);
#13077=AXIS2_PLACEMENT_3D('',#20053,#15725,#15726);
#13078=AXIS2_PLACEMENT_3D('',#20054,#15727,#15728);
#13079=AXIS2_PLACEMENT_3D('',#20067,#15735,#15736);
#13080=AXIS2_PLACEMENT_3D('',#20073,#15740,#15741);
#13081=AXIS2_PLACEMENT_3D('',#20077,#15744,#15745);
#13082=AXIS2_PLACEMENT_3D('',#20081,#15748,#15749);
#13083=AXIS2_PLACEMENT_3D('',#20085,#15752,#15753);
#13084=AXIS2_PLACEMENT_3D('',#20089,#15756,#15757);
#13085=AXIS2_PLACEMENT_3D('',#20091,#15759,#15760);
#13086=AXIS2_PLACEMENT_3D('',#20104,#15767,#15768);
#13087=AXIS2_PLACEMENT_3D('',#20118,#15776,#15777);
#13088=AXIS2_PLACEMENT_3D('',#20126,#15783,#15784);
#13089=AXIS2_PLACEMENT_3D('',#20128,#15786,#15787);
#13090=AXIS2_PLACEMENT_3D('',#20130,#15789,#15790);
#13091=AXIS2_PLACEMENT_3D('',#20131,#15791,#15792);
#13092=AXIS2_PLACEMENT_3D('',#20135,#15794,#15795);
#13093=AXIS2_PLACEMENT_3D('',#20137,#15797,#15798);
#13094=AXIS2_PLACEMENT_3D('',#20141,#15801,#15802);
#13095=AXIS2_PLACEMENT_3D('',#20144,#15804,#15805);
#13096=AXIS2_PLACEMENT_3D('',#20145,#15806,#15807);
#13097=AXIS2_PLACEMENT_3D('',#20147,#15809,#15810);
#13098=AXIS2_PLACEMENT_3D('',#20151,#15813,#15814);
#13099=AXIS2_PLACEMENT_3D('',#20155,#15817,#15818);
#13100=AXIS2_PLACEMENT_3D('',#20159,#15821,#15822);
#13101=AXIS2_PLACEMENT_3D('',#20163,#15825,#15826);
#13102=AXIS2_PLACEMENT_3D('',#20167,#15829,#15830);
#13103=AXIS2_PLACEMENT_3D('',#20171,#15833,#15834);
#13104=AXIS2_PLACEMENT_3D('',#20175,#15836,#15837);
#13105=AXIS2_PLACEMENT_3D('',#20178,#15840,#15841);
#13106=AXIS2_PLACEMENT_3D('',#20183,#15844,#15845);
#13107=AXIS2_PLACEMENT_3D('',#20184,#15846,#15847);
#13108=AXIS2_PLACEMENT_3D('',#20188,#15849,#15850);
#13109=AXIS2_PLACEMENT_3D('',#20191,#15852,#15853);
#13110=AXIS2_PLACEMENT_3D('',#20192,#15854,#15855);
#13111=AXIS2_PLACEMENT_3D('',#20195,#15857,#15858);
#13112=AXIS2_PLACEMENT_3D('',#20197,#15860,#15861);
#13113=AXIS2_PLACEMENT_3D('',#20201,#15863,#15864);
#13114=AXIS2_PLACEMENT_3D('',#20203,#15866,#15867);
#13115=AXIS2_PLACEMENT_3D('',#20205,#15868,#15869);
#13116=AXIS2_PLACEMENT_3D('',#20208,#15871,#15872);
#13117=AXIS2_PLACEMENT_3D('',#20209,#15873,#15874);
#13118=AXIS2_PLACEMENT_3D('',#20211,#15875,#15876);
#13119=AXIS2_PLACEMENT_3D('',#20212,#15877,#15878);
#13120=AXIS2_PLACEMENT_3D('',#20214,#15879,#15880);
#13121=AXIS2_PLACEMENT_3D('',#20215,#15881,#15882);
#13122=AXIS2_PLACEMENT_3D('',#20216,#15883,#15884);
#13123=AXIS2_PLACEMENT_3D('',#20218,#15886,#15887);
#13124=AXIS2_PLACEMENT_3D('',#20220,#15889,#15890);
#13125=AXIS2_PLACEMENT_3D('',#20224,#15893,#15894);
#13126=AXIS2_PLACEMENT_3D('',#20228,#15897,#15898);
#13127=AXIS2_PLACEMENT_3D('',#20230,#15900,#15901);
#13128=AXIS2_PLACEMENT_3D('',#20232,#15903,#15904);
#13129=AXIS2_PLACEMENT_3D('',#20233,#15905,#15906);
#13130=AXIS2_PLACEMENT_3D('',#20234,#15907,#15908);
#13131=AXIS2_PLACEMENT_3D('',#20235,#15909,#15910);
#13132=AXIS2_PLACEMENT_3D('',#20236,#15911,#15912);
#13133=AXIS2_PLACEMENT_3D('',#20237,#15913,#15914);
#13134=AXIS2_PLACEMENT_3D('',#20238,#15915,#15916);
#13135=AXIS2_PLACEMENT_3D('',#20330,#15919,#15920);
#13136=AXIS2_PLACEMENT_3D('',#20425,#15923,#15924);
#13137=AXIS2_PLACEMENT_3D('',#20426,#15925,#15926);
#13138=AXIS2_PLACEMENT_3D('',#20427,#15927,#15928);
#13139=AXIS2_PLACEMENT_3D('',#20428,#15929,#15930);
#13140=AXIS2_PLACEMENT_3D('',#20583,#15931,#15932);
#13141=AXIS2_PLACEMENT_3D('',#20638,#15933,#15934);
#13142=AXIS2_PLACEMENT_3D('',#20639,#15935,#15936);
#13143=AXIS2_PLACEMENT_3D('',#20767,#15937,#15938);
#13144=AXIS2_PLACEMENT_3D('',#20768,#15939,#15940);
#13145=AXIS2_PLACEMENT_3D('',#20769,#15941,#15942);
#13146=AXIS2_PLACEMENT_3D('',#20770,#15943,#15944);
#13147=AXIS2_PLACEMENT_3D('',#20771,#15945,#15946);
#13148=AXIS2_PLACEMENT_3D('',#20772,#15947,#15948);
#13149=AXIS2_PLACEMENT_3D('',#21012,#15949,#15950);
#13150=AXIS2_PLACEMENT_3D('',#21049,#15951,#15952);
#13151=AXIS2_PLACEMENT_3D('',#21116,#15953,#15954);
#13152=AXIS2_PLACEMENT_3D('',#21117,#15955,#15956);
#13153=AXIS2_PLACEMENT_3D('',#21118,#15957,#15958);
#13154=AXIS2_PLACEMENT_3D('',#21119,#15959,#15960);
#13155=AXIS2_PLACEMENT_3D('',#21120,#15961,#15962);
#13156=AXIS2_PLACEMENT_3D('',#21121,#15963,#15964);
#13157=AXIS2_PLACEMENT_3D('',#21122,#15965,#15966);
#13158=AXIS2_PLACEMENT_3D('',#21123,#15967,#15968);
#13159=AXIS2_PLACEMENT_3D('',#21124,#15969,#15970);
#13160=AXIS2_PLACEMENT_3D('',#21125,#15971,#15972);
#13161=AXIS2_PLACEMENT_3D('',#21126,#15973,#15974);
#13162=AXIS2_PLACEMENT_3D('',#21127,#15975,#15976);
#13163=AXIS2_PLACEMENT_3D('',#21128,#15977,#15978);
#15530=DIRECTION('axis',(0.,0.,1.));
#15531=DIRECTION('refdir',(1.,0.,0.));
#15532=DIRECTION('center_axis',(-0.974431531646231,0.224684645967589,-1.26428912495664E-17));
#15533=DIRECTION('ref_axis',(-1.23196318847518E-17,2.84066354441556E-18,
1.));
#15534=DIRECTION('',(-0.974431531646231,0.224684645967589,-1.26428912495664E-17));
#15535=DIRECTION('center_axis',(-0.974431531646231,0.224684645967589,-1.26428912495664E-17));
#15536=DIRECTION('ref_axis',(-1.23196318847518E-17,2.84066354441556E-18,
1.));
#15537=DIRECTION('center_axis',(2.08745462991212E-17,1.24347063228184E-16,
-1.));
#15538=DIRECTION('ref_axis',(-0.974431531646231,0.22468464596759,0.));
#15539=DIRECTION('center_axis',(2.08745462991212E-17,1.24347063228184E-16,
-1.));
#15540=DIRECTION('ref_axis',(-0.974431531646231,0.224684645967589,7.59805975586113E-18));
#15541=DIRECTION('center_axis',(-0.224684645967589,-0.974431531646231,-1.25857889322102E-16));
#15542=DIRECTION('ref_axis',(0.974431531646231,-0.224684645967589,0.));
#15543=DIRECTION('center_axis',(-2.08745462991212E-17,-1.24347063228184E-16,
1.));
#15544=DIRECTION('ref_axis',(-0.974431531646231,0.224684645967589,7.59805975586113E-18));
#15545=DIRECTION('center_axis',(-2.08745462991212E-17,-1.24347063228184E-16,
1.));
#15546=DIRECTION('ref_axis',(-0.974431531646231,0.224684645967589,7.59805975586113E-18));
#15547=DIRECTION('center_axis',(2.08745462991212E-17,1.24347063228184E-16,
-1.));
#15548=DIRECTION('ref_axis',(-0.974431531646231,0.22468464596759,0.));
#15549=DIRECTION('center_axis',(2.08745462991212E-17,1.24347063228184E-16,
-1.));
#15550=DIRECTION('ref_axis',(-0.974431531646231,0.224684645967589,7.59805975586113E-18));
#15551=DIRECTION('center_axis',(2.08745462991212E-17,1.24347063228184E-16,
-1.));
#15552=DIRECTION('ref_axis',(-0.974431531646231,0.224684645967589,7.59805975586113E-18));
#15553=DIRECTION('center_axis',(-0.224684645967589,-0.974431531646231,-1.25857889322102E-16));
#15554=DIRECTION('ref_axis',(0.974431531646231,-0.224684645967589,0.));
#15555=DIRECTION('center_axis',(-2.08745462991212E-17,-1.24347063228184E-16,
1.));
#15556=DIRECTION('ref_axis',(-0.974431531646231,0.224684645967589,7.59805975586113E-18));
#15557=DIRECTION('center_axis',(-0.974431531646231,0.224684645967589,-1.26428912495664E-17));
#15558=DIRECTION('ref_axis',(-1.23196318847518E-17,2.84066354441556E-18,
1.));
#15559=DIRECTION('center_axis',(-0.974431531646231,0.224684645967589,-1.26428912495664E-17));
#15560=DIRECTION('ref_axis',(-1.23196318847518E-17,2.84066354441556E-18,
1.));
#15561=DIRECTION('',(-0.974431531646231,0.224684645967589,-1.26428912495664E-17));
#15562=DIRECTION('center_axis',(-0.974431531646231,0.224684645967589,-1.26428912495664E-17));
#15563=DIRECTION('ref_axis',(-1.23196318847518E-17,2.84066354441556E-18,
1.));
#15564=DIRECTION('center_axis',(0.224684645967589,0.974431531646231,6.60780807231409E-17));
#15565=DIRECTION('ref_axis',(1.48467301734967E-17,6.43885654072935E-17,
-1.));
#15566=DIRECTION('center_axis',(0.224684645967589,0.974431531646231,6.60780807231409E-17));
#15567=DIRECTION('ref_axis',(1.48467301734967E-17,6.43885654072935E-17,
-1.));
#15568=DIRECTION('',(0.224684645967589,0.974431531646231,6.60780807231409E-17));
#15569=DIRECTION('center_axis',(0.224684645967589,0.974431531646231,6.60780807231409E-17));
#15570=DIRECTION('ref_axis',(1.48467301734967E-17,6.43885654072935E-17,
-1.));
#15571=DIRECTION('center_axis',(2.08745462991212E-17,1.24347063228184E-16,
-1.));
#15572=DIRECTION('ref_axis',(-0.974431531646231,0.224684645967588,7.59805975586093E-18));
#15573=DIRECTION('center_axis',(2.08745462991212E-17,1.24347063228184E-16,
-1.));
#15574=DIRECTION('ref_axis',(-0.974431531646231,0.224684645967588,7.59805975586093E-18));
#15575=DIRECTION('',(2.08745462991212E-17,1.24347063228184E-16,-1.));
#15576=DIRECTION('center_axis',(2.08745462991212E-17,1.24347063228184E-16,
-1.));
#15577=DIRECTION('ref_axis',(-0.974431531646231,0.224684645967588,7.59805975586093E-18));
#15578=DIRECTION('center_axis',(2.08745462991212E-17,1.24347063228184E-16,
-1.));
#15579=DIRECTION('ref_axis',(-0.974431531646231,0.224684645967589,7.59805975586113E-18));
#15580=DIRECTION('center_axis',(2.08745462991212E-17,1.24347063228184E-16,
-1.));
#15581=DIRECTION('ref_axis',(-0.974431531646231,0.224684645967589,7.59805975586113E-18));
#15582=DIRECTION('',(2.08745462991212E-17,1.24347063228184E-16,-1.));
#15583=DIRECTION('center_axis',(2.08745462991212E-17,1.24347063228184E-16,
-1.));
#15584=DIRECTION('ref_axis',(-0.974431531646231,0.224684645967589,7.59805975586113E-18));
#15585=DIRECTION('center_axis',(-0.147090628234403,-0.637915179045802,0.755928946018455));
#15586=DIRECTION('ref_axis',(0.169845627612808,0.736601000684484,0.654653670707977));
#15587=DIRECTION('center_axis',(0.224684645967553,0.974431531646239,-1.2074073682481E-13));
#15588=DIRECTION('ref_axis',(-2.27979080437047E-11,5.38065576097235E-12,
1.));
#15589=DIRECTION('center_axis',(-0.843882460965992,0.194582612535136,-0.499999998972983));
#15590=DIRECTION('ref_axis',(0.50338836685051,0.609594266156192,-0.612368339146523));
#15591=DIRECTION('',(0.147090628234403,0.637915179045802,-0.755928946018455));
#15592=DIRECTION('center_axis',(-0.48721576582319,0.112342322983636,0.866025403784417));
#15593=DIRECTION('ref_axis',(0.227358619108416,-0.941173766267205,0.250000000015036));
#15594=DIRECTION('center_axis',(0.487215765823101,-0.11234232298411,0.866025403784406));
#15595=DIRECTION('ref_axis',(-0.616523841550484,-0.746591155056556,0.249999999982304));
#15596=DIRECTION('',(-0.147090628234403,-0.637915179045802,0.755928946018454));
#15597=DIRECTION('center_axis',(-0.843882461168241,0.19458261062525,0.499999999374895));
#15598=DIRECTION('ref_axis',(0.185637904156542,-0.768464715336596,0.612372884624238));
#15599=DIRECTION('center_axis',(0.147090628234407,0.637915179045802,0.755928946018454));
#15600=DIRECTION('ref_axis',(0.169845627612808,0.736601000684483,-0.654653670707978));
#15601=DIRECTION('center_axis',(0.487215765823114,-0.112342322983753,-0.866025403784445));
#15602=DIRECTION('ref_axis',(0.616523841554425,0.746591155052271,0.249999999985382));
#15603=DIRECTION('center_axis',(-0.487215765823237,0.11234232298353,-0.866025403784404));
#15604=DIRECTION('ref_axis',(-0.227358619080957,0.94117376627761,0.250000000000839));
#15605=DIRECTION('',(-0.147090628234407,-0.637915179045802,-0.755928946018454));
#15606=DIRECTION('center_axis',(-0.843882459372318,0.194582605937149,0.500000004230436));
#15607=DIRECTION('ref_axis',(0.503389000994448,0.60959164109859,0.612370431014218));
#15608=DIRECTION('center_axis',(0.224684645967565,0.974431531646236,6.66256114045275E-14));
#15609=DIRECTION('ref_axis',(6.59444949636519E-12,-1.58892350212702E-12,
1.));
#15610=DIRECTION('center_axis',(-0.843882462501695,0.194582609008347,-0.499999997753581));
#15611=DIRECTION('ref_axis',(-0.18563903427446,0.768463346797486,0.612374259405515));
#15612=DIRECTION('',(0.147090628234407,0.637915179045802,0.755928946018454));
#15613=DIRECTION('center_axis',(-0.224684645967589,-0.974431531646231,-6.60780807231409E-17));
#15614=DIRECTION('ref_axis',(-0.974431531646231,0.224684645967589,-3.69778549322349E-32));
#15615=DIRECTION('center_axis',(0.224684645967589,0.974431531646231,6.60780807231409E-17));
#15616=DIRECTION('ref_axis',(-0.974431531646231,0.224684645967589,-3.69778549322349E-32));
#15617=DIRECTION('',(0.224684645967589,0.974431531646231,6.60780807231409E-17));
#15618=DIRECTION('center_axis',(0.224684645967589,0.974431531646231,6.60780807231409E-17));
#15619=DIRECTION('ref_axis',(0.974431531646231,-0.224684645967589,3.69778549322349E-32));
#15620=DIRECTION('center_axis',(0.224684645967589,0.974431531646231,6.60780807231409E-17));
#15621=DIRECTION('ref_axis',(0.974431531646231,-0.224684645967589,3.69778549322349E-32));
#15622=DIRECTION('center_axis',(0.224684645967589,0.974431531646231,6.60780807231409E-17));
#15623=DIRECTION('ref_axis',(0.974431531646231,-0.224684645967589,3.69778549322349E-32));
#15624=DIRECTION('center_axis',(0.224684645967589,0.974431531646231,6.60780807231409E-17));
#15625=DIRECTION('ref_axis',(0.974431531646231,-0.224684645967589,3.69778549322349E-32));
#15626=DIRECTION('center_axis',(0.224684645967589,0.974431531646231,6.60780807231409E-17));
#15627=DIRECTION('ref_axis',(0.974431531646231,-0.224684645967589,3.69778549322349E-32));
#15628=DIRECTION('center_axis',(0.224684645967589,0.974431531646231,6.60780807231409E-17));
#15629=DIRECTION('ref_axis',(0.974431531646231,-0.224684645967589,3.69778549322349E-32));
#15630=DIRECTION('center_axis',(9.84588993227597E-17,-1.5186299647836E-16,
1.));
#15631=DIRECTION('ref_axis',(0.974431531646231,-0.224684645967587,-1.30062739670596E-16));
#15632=DIRECTION('center_axis',(8.84893164462714E-17,1.08756434026123E-16,
-1.));
#15633=DIRECTION('ref_axis',(0.974431531646231,-0.22468464596759,6.17908792832111E-17));
#15634=DIRECTION('',(-9.84588993227597E-17,1.5186299647836E-16,-1.));
#15635=DIRECTION('center_axis',(-2.08745462991212E-17,-1.24347063228184E-16,
1.));
#15636=DIRECTION('ref_axis',(-0.974431531646223,0.224684645967624,7.59805975586562E-18));
#15637=DIRECTION('',(9.84588993227597E-17,-1.5186299647836E-16,1.));
#15638=DIRECTION('center_axis',(-0.974431531646231,0.224684645967589,-1.26428912495664E-17));
#15639=DIRECTION('ref_axis',(0.224684645967589,0.974431531646231,-2.31111593326468E-33));
#15640=DIRECTION('center_axis',(-0.974431531646231,0.224684645967589,-1.26428912495664E-17));
#15641=DIRECTION('ref_axis',(0.224684645967589,0.974431531646231,-2.31111593326468E-33));
#15642=DIRECTION('',(0.974431531646231,-0.224684645967589,1.26428912495664E-17));
#15643=DIRECTION('center_axis',(-0.974431531646231,0.224684645967589,-1.26428912495664E-17));
#15644=DIRECTION('ref_axis',(0.224684645967589,0.974431531646231,-2.31111593326468E-33));
#15645=DIRECTION('center_axis',(-0.974431531646231,0.224684645967589,-1.26428912495664E-17));
#15646=DIRECTION('ref_axis',(0.224684645967589,0.974431531646231,-2.69630192214213E-33));
#15647=DIRECTION('center_axis',(-0.974431531646231,0.224684645967589,-1.26428912495664E-17));
#15648=DIRECTION('ref_axis',(0.224684645967589,0.974431531646231,-2.69630192214213E-33));
#15649=DIRECTION('',(0.974431531646231,-0.224684645967589,1.26428912495664E-17));
#15650=DIRECTION('center_axis',(-0.974431531646231,0.224684645967589,-1.26428912495664E-17));
#15651=DIRECTION('ref_axis',(0.224684645967589,0.974431531646231,-2.69630192214213E-33));
#15652=DIRECTION('center_axis',(-0.974431531646231,0.224684645967589,-1.26428912495664E-17));
#15653=DIRECTION('ref_axis',(0.224684645967589,0.974431531646231,-2.31111593326468E-33));
#15654=DIRECTION('center_axis',(-0.974431531646231,0.224684645967589,-1.26428912495664E-17));
#15655=DIRECTION('ref_axis',(0.224684645967589,0.974431531646231,-2.31111593326468E-33));
#15656=DIRECTION('',(0.974431531646231,-0.224684645967589,1.26428912495664E-17));
#15657=DIRECTION('center_axis',(-0.974431531646231,0.224684645967589,-1.26428912495664E-17));
#15658=DIRECTION('ref_axis',(0.224684645967589,0.974431531646231,-1.15555796663234E-33));
#15659=DIRECTION('center_axis',(-0.974431531646231,0.224684645967589,-1.26428912495664E-17));
#15660=DIRECTION('ref_axis',(0.224684645967589,0.974431531646231,-3.85185988877447E-34));
#15661=DIRECTION('center_axis',(-0.974431531646231,0.224684645967589,-1.26428912495664E-17));
#15662=DIRECTION('ref_axis',(0.224684645967589,0.974431531646231,-3.85185988877447E-34));
#15663=DIRECTION('',(0.974431531646231,-0.224684645967589,1.26428912495664E-17));
#15664=DIRECTION('center_axis',(-0.974431531646231,0.224684645967589,-1.26428912495664E-17));
#15665=DIRECTION('ref_axis',(0.224684645967589,0.974431531646231,-3.85185988877447E-34));
#15666=DIRECTION('center_axis',(-0.974431531646231,0.224684645967589,-1.26428912495664E-17));
#15667=DIRECTION('ref_axis',(0.224684645967589,0.974431531646231,-3.85185988877447E-34));
#15668=DIRECTION('center_axis',(-0.974431531646231,0.224684645967589,-1.26428912495664E-17));
#15669=DIRECTION('ref_axis',(0.224684645967589,0.974431531646231,-3.85185988877447E-34));
#15670=DIRECTION('center_axis',(-0.974431531646231,0.224684645967589,-1.26428912495664E-17));
#15671=DIRECTION('ref_axis',(0.224684645967589,0.974431531646231,-3.85185988877447E-34));
#15672=DIRECTION('center_axis',(-0.94183030799337,0.336088784319134,1.16739108769533E-16));
#15673=DIRECTION('ref_axis',(-0.336088784319135,-0.94183030799337,-6.36115566062716E-14));
#15674=DIRECTION('',(0.997691327175712,-0.0679118228172861,-6.86415162287128E-18));
#15675=DIRECTION('center_axis',(-0.974431531646231,0.224684645967589,-1.26428912495664E-17));
#15676=DIRECTION('ref_axis',(0.224684645967589,0.974431531646231,-2.31111593326468E-33));
#15677=DIRECTION('center_axis',(-0.974431531646231,0.224684645967589,-1.26428912495664E-17));
#15678=DIRECTION('ref_axis',(0.224684645967589,0.974431531646231,-2.31111593326468E-33));
#15679=DIRECTION('center_axis',(-0.974431531646231,0.224684645967589,-1.26428912495664E-17));
#15680=DIRECTION('ref_axis',(0.224684645967589,0.974431531646231,-2.31111593326468E-33));
#15681=DIRECTION('center_axis',(-0.974431531646231,0.224684645967589,-1.26428912495664E-17));
#15682=DIRECTION('ref_axis',(0.224684645967589,0.974431531646231,-2.31111593326468E-33));
#15683=DIRECTION('center_axis',(-0.974431531646231,0.224684645967589,-1.26428912495664E-17));
#15684=DIRECTION('ref_axis',(0.224684645967589,0.974431531646231,-2.31111593326468E-33));
#15685=DIRECTION('center_axis',(-2.08745462991212E-17,-1.24347063228184E-16,
1.));
#15686=DIRECTION('ref_axis',(0.974431531646231,-0.224684645967589,-7.59805975586113E-18));
#15687=DIRECTION('',(2.08745462991212E-17,1.24347063228184E-16,-1.));
#15688=DIRECTION('',(2.08745462991212E-17,1.24347063228184E-16,-1.));
#15689=DIRECTION('',(2.08745462991212E-17,1.24347063228184E-16,-1.));
#15690=DIRECTION('',(-2.08745462991212E-17,-1.24347063228184E-16,1.));
#15691=DIRECTION('center_axis',(-0.224684645967589,-0.974431531646231,-6.60780807231409E-17));
#15692=DIRECTION('ref_axis',(-0.974431531646231,0.224684645967589,-1.26428912495664E-17));
#15693=DIRECTION('',(-2.08745462991212E-17,-1.24347063228184E-16,1.));
#15694=DIRECTION('',(0.974431531646231,-0.224684645967589,1.26428912495664E-17));
#15695=DIRECTION('',(2.08745462991212E-17,1.24347063228184E-16,-1.));
#15696=DIRECTION('',(-0.974431531646231,0.224684645967589,-1.26428912495664E-17));
#15697=DIRECTION('center_axis',(2.08745462991212E-17,1.24347063228184E-16,
-1.));
#15698=DIRECTION('ref_axis',(-0.974431531646231,0.224684645967589,7.59805975586114E-18));
#15699=DIRECTION('',(2.08745462991212E-17,1.24347063228184E-16,-1.));
#15700=DIRECTION('center_axis',(0.224684645967589,0.974431531646231,6.60780807231409E-17));
#15701=DIRECTION('ref_axis',(0.974431531646231,-0.224684645967589,1.26428912495664E-17));
#15702=DIRECTION('',(2.08745462991212E-17,1.24347063228184E-16,-1.));
#15703=DIRECTION('',(0.974431531646231,-0.224684645967589,1.26428912495664E-17));
#15704=DIRECTION('',(-0.974431531646231,0.224684645967589,-1.26428912495664E-17));
#15705=DIRECTION('center_axis',(4.05979671893162E-17,1.19799232317482E-16,
-1.));
#15706=DIRECTION('ref_axis',(-0.974431531646231,0.224684645967589,-1.26428912495664E-17));
#15707=DIRECTION('center_axis',(4.05979671893162E-17,1.19799232317482E-16,
-1.));
#15708=DIRECTION('ref_axis',(-0.974431531646231,0.224684645967589,-1.26428912495664E-17));
#15709=DIRECTION('center_axis',(0.974431531646231,-0.224684645967589,1.26428912495664E-17));
#15710=DIRECTION('ref_axis',(-0.224684645967589,-0.974431531646231,-6.60780807231409E-17));
#15711=DIRECTION('center_axis',(-0.974431531646231,0.224684645967589,-1.26428912495664E-17));
#15712=DIRECTION('ref_axis',(-0.224684645967589,-0.974431531646231,-1.42518815884655E-32));
#15713=DIRECTION('center_axis',(-0.974431531646231,0.224684645967589,-1.26428912495664E-17));
#15714=DIRECTION('ref_axis',(-0.224684645967589,-0.974431531646231,-1.42518815884655E-32));
#15715=DIRECTION('center_axis',(0.974431531646231,-0.224684645967589,1.26428912495664E-17));
#15716=DIRECTION('ref_axis',(-0.224684645967589,-0.974431531646231,-6.60780807231409E-17));
#15717=DIRECTION('center_axis',(-0.974431531646231,0.224684645967589,-1.26428912495664E-17));
#15718=DIRECTION('ref_axis',(-0.224684645967589,-0.974431531646231,1.38777878078144E-14));
#15719=DIRECTION('center_axis',(-0.974431531646231,0.224684645967589,-1.26428912495664E-17));
#15720=DIRECTION('ref_axis',(-0.224684645967589,-0.974431531646231,-1.42518815884655E-32));
#15721=DIRECTION('center_axis',(-0.974431531646231,0.224684645967589,-1.26428912495664E-17));
#15722=DIRECTION('ref_axis',(0.224684645967589,0.974431531646231,6.60780807231409E-17));
#15723=DIRECTION('center_axis',(-0.974431531646231,0.224684645967589,-1.26428912495664E-17));
#15724=DIRECTION('ref_axis',(0.224684645967589,0.974431531646231,6.60780807231409E-17));
#15725=DIRECTION('center_axis',(-0.974431531646231,0.224684645967589,-1.26428912495664E-17));
#15726=DIRECTION('ref_axis',(0.224684645967589,0.974431531646231,6.60780807231409E-17));
#15727=DIRECTION('center_axis',(-0.974431531646231,0.224684645967589,-1.26428912495664E-17));
#15728=DIRECTION('ref_axis',(0.224684645967589,0.974431531646231,6.60780807231409E-17));
#15729=DIRECTION('',(0.112342322983794,0.487215765823115,-0.866025403784439));
#15730=DIRECTION('',(0.224684645967589,0.974431531646231,-9.52915449491201E-17));
#15731=DIRECTION('',(0.112342322983794,0.487215765823115,0.866025403784438));
#15732=DIRECTION('',(-0.112342322983794,-0.487215765823116,0.866025403784438));
#15733=DIRECTION('',(-0.224684645967589,-0.974431531646231,2.56661170621381E-16));
#15734=DIRECTION('',(-0.112342322983794,-0.487215765823116,-0.866025403784438));
#15735=DIRECTION('center_axis',(-0.194582611248245,-0.843882460654216,-0.5));
#15736=DIRECTION('ref_axis',(-0.112342322983794,-0.487215765823115,0.866025403784439));
#15737=DIRECTION('',(0.974431531646231,-0.224684645967589,1.26428912495664E-17));
#15738=DIRECTION('',(-0.112342322983794,-0.487215765823115,0.866025403784439));
#15739=DIRECTION('',(0.974431531646231,-0.224684645967589,1.26428912495664E-17));
#15740=DIRECTION('center_axis',(-0.194582611248245,-0.843882460654216,0.5));
#15741=DIRECTION('ref_axis',(0.112342322983794,0.487215765823116,0.866025403784438));
#15742=DIRECTION('',(0.974431531646231,-0.224684645967589,1.26428912495664E-17));
#15743=DIRECTION('',(0.112342322983794,0.487215765823116,0.866025403784438));
#15744=DIRECTION('center_axis',(6.50716132601352E-17,2.48391570236421E-16,
1.));
#15745=DIRECTION('ref_axis',(0.224684645967589,0.974431531646231,-2.56661170621381E-16));
#15746=DIRECTION('',(0.974431531646231,-0.224684645967589,1.26428912495664E-17));
#15747=DIRECTION('',(0.224684645967589,0.974431531646231,-2.56661170621381E-16));
#15748=DIRECTION('center_axis',(0.194582611248245,0.843882460654216,0.5));
#15749=DIRECTION('ref_axis',(0.112342322983794,0.487215765823116,-0.866025403784439));
#15750=DIRECTION('',(0.974431531646231,-0.224684645967589,1.26428912495664E-17));
#15751=DIRECTION('',(0.112342322983794,0.487215765823116,-0.866025403784438));
#15752=DIRECTION('center_axis',(0.194582611248245,0.843882460654216,-0.5));
#15753=DIRECTION('ref_axis',(-0.112342322983794,-0.487215765823116,-0.866025403784439));
#15754=DIRECTION('',(0.974431531646231,-0.224684645967589,1.26428912495664E-17));
#15755=DIRECTION('',(-0.112342322983794,-0.487215765823116,-0.866025403784438));
#15756=DIRECTION('center_axis',(-2.88143360460409E-17,-9.11479187314206E-17,
-1.));
#15757=DIRECTION('ref_axis',(-0.224684645967589,-0.974431531646231,9.52915449491202E-17));
#15758=DIRECTION('',(-0.224684645967589,-0.974431531646231,9.52915449491202E-17));
#15759=DIRECTION('center_axis',(-0.974431531646231,0.224684645967589,7.59805975586106E-18));
#15760=DIRECTION('ref_axis',(-2.08745462991212E-17,-1.24347063228184E-16,
1.));
#15761=DIRECTION('',(0.112342322983794,0.487215765823116,0.866025403784438));
#15762=DIRECTION('',(0.224684645967589,0.974431531646231,-9.52915449491202E-17));
#15763=DIRECTION('',(0.112342322983794,0.487215765823115,-0.866025403784439));
#15764=DIRECTION('',(-0.112342322983794,-0.487215765823116,-0.866025403784438));
#15765=DIRECTION('',(-0.224684645967589,-0.974431531646231,2.56661170621381E-16));
#15766=DIRECTION('',(-0.112342322983794,-0.487215765823116,0.866025403784438));
#15767=DIRECTION('center_axis',(0.224684645967589,0.974431531646231,1.25857889322102E-16));
#15768=DIRECTION('ref_axis',(2.08745462991212E-17,1.24347063228184E-16,
-1.));
#15769=DIRECTION('',(-0.974431531646231,0.224684645967589,1.09821788665169E-16));
#15770=DIRECTION('',(2.08745462991212E-17,1.24347063228184E-16,-1.));
#15771=DIRECTION('',(0.974431531646231,-0.224684645967589,1.26428912495664E-17));
#15772=DIRECTION('',(0.,0.,1.));
#15773=DIRECTION('',(0.974431531646231,-0.224684645967588,0.));
#15774=DIRECTION('',(-0.974431531646231,0.224684645967588,0.));
#15775=DIRECTION('',(0.,0.,1.));
#15776=DIRECTION('center_axis',(0.974431531646231,-0.224684645967589,-7.59805975586106E-18));
#15777=DIRECTION('ref_axis',(2.08745462991212E-17,1.24347063228184E-16,
-1.));
#15778=DIRECTION('',(0.224684645967589,0.974431531646231,6.60780807231409E-17));
#15779=DIRECTION('',(-0.224684645967589,-0.974431531646231,-6.60780807231409E-17));
#15780=DIRECTION('',(-2.08745462991212E-17,-1.24347063228184E-16,1.));
#15781=DIRECTION('',(-0.224684645967589,-0.974431531646231,-6.60780807231409E-17));
#15782=DIRECTION('',(0.224684645967589,0.974431531646231,6.60780807231409E-17));
#15783=DIRECTION('center_axis',(-1.08212737336466E-16,-1.04208603115422E-16,
1.));
#15784=DIRECTION('ref_axis',(0.974431531646231,-0.224684645967589,8.20318302886387E-17));
#15785=DIRECTION('',(0.336088784319134,0.94183030799337,9.58152703863411E-17));
#15786=DIRECTION('center_axis',(4.05979671893162E-17,1.19799232317482E-16,
-1.));
#15787=DIRECTION('ref_axis',(-0.974431531646231,0.224684645967589,-1.26428912495664E-17));
#15788=DIRECTION('',(0.336088784319134,0.94183030799337,6.70979889663902E-17));
#15789=DIRECTION('center_axis',(-0.94183030799337,0.336088784319134,1.16739108769533E-16));
#15790=DIRECTION('ref_axis',(0.336088784319134,0.94183030799337,6.70979889663902E-17));
#15791=DIRECTION('center_axis',(4.05979671893162E-17,1.19799232317482E-16,
-1.));
#15792=DIRECTION('ref_axis',(-0.974431531646231,0.224684645967589,-1.26428912495664E-17));
#15793=DIRECTION('',(-0.224684645967589,-0.974431531646231,-6.60780807231409E-17));
#15794=DIRECTION('center_axis',(-2.08745462991212E-17,-1.24347063228184E-16,
1.));
#15795=DIRECTION('ref_axis',(-0.974431531646231,0.224684645967587,7.59805975586085E-18));
#15796=DIRECTION('',(0.974431531646231,-0.224684645967589,1.26428912495664E-17));
#15797=DIRECTION('center_axis',(-0.974431531646231,0.224684645967589,7.59805975586106E-18));
#15798=DIRECTION('ref_axis',(-2.08745462991212E-17,-1.24347063228184E-16,
1.));
#15799=DIRECTION('',(-0.224684645967589,-0.974431531646231,-6.60780807231409E-17));
#15800=DIRECTION('',(-2.08745462991212E-17,-1.24347063228184E-16,1.));
#15801=DIRECTION('center_axis',(7.87354784325647E-17,-1.47315165567658E-16,
1.));
#15802=DIRECTION('ref_axis',(0.974431531646231,-0.224684645967589,-1.09821788665169E-16));
#15803=DIRECTION('',(-0.974431531646231,0.224684645967589,1.09821788665169E-16));
#15804=DIRECTION('center_axis',(-9.84588993227598E-17,1.5186299647836E-16,
-1.));
#15805=DIRECTION('ref_axis',(0.974431531646237,-0.224684645967561,-1.30062739670593E-16));
#15806=DIRECTION('center_axis',(-0.224684645967589,-0.974431531646231,-1.25857889322102E-16));
#15807=DIRECTION('ref_axis',(-2.08745462991212E-17,-1.24347063228184E-16,
1.));
#15808=DIRECTION('',(2.08745462991212E-17,1.24347063228184E-16,-1.));
#15809=DIRECTION('center_axis',(0.224684645967589,0.974431531646231,1.25857889322102E-16));
#15810=DIRECTION('ref_axis',(2.08745462991212E-17,1.24347063228184E-16,
-1.));
#15811=DIRECTION('',(-3.69499511157397E-16,2.14359602894637E-16,-1.));
#15812=DIRECTION('',(-0.843882460654216,0.194582611248245,-0.5));
#15813=DIRECTION('center_axis',(0.224684645967589,0.974431531646231,1.25857889322102E-16));
#15814=DIRECTION('ref_axis',(2.08745462991212E-17,1.24347063228184E-16,
-1.));
#15815=DIRECTION('',(-0.843882460654216,0.194582611248245,-0.5));
#15816=DIRECTION('',(-0.843882460654216,0.194582611248245,0.5));
#15817=DIRECTION('center_axis',(0.224684645967589,0.974431531646231,1.25857889322102E-16));
#15818=DIRECTION('ref_axis',(2.08745462991212E-17,1.24347063228184E-16,
-1.));
#15819=DIRECTION('',(-0.843882460654216,0.194582611248245,0.5));
#15820=DIRECTION('',(-1.18468060663251E-16,-1.01843928311571E-16,1.));
#15821=DIRECTION('center_axis',(0.224684645967589,0.974431531646231,1.25857889322102E-16));
#15822=DIRECTION('ref_axis',(2.08745462991212E-17,1.24347063228184E-16,
-1.));
#15823=DIRECTION('',(-1.18468060663251E-16,-1.01843928311571E-16,1.));
#15824=DIRECTION('',(0.843882460654216,-0.194582611248245,0.5));
#15825=DIRECTION('center_axis',(0.224684645967589,0.974431531646231,1.25857889322102E-16));
#15826=DIRECTION('ref_axis',(2.08745462991212E-17,1.24347063228184E-16,
-1.));
#15827=DIRECTION('',(0.843882460654216,-0.194582611248245,0.5));
#15828=DIRECTION('',(0.843882460654216,-0.194582611248245,-0.5));
#15829=DIRECTION('center_axis',(0.224684645967589,0.974431531646231,1.25857889322102E-16));
#15830=DIRECTION('ref_axis',(2.08745462991212E-17,1.24347063228184E-16,
-1.));
#15831=DIRECTION('',(0.843882460654216,-0.194582611248245,-0.5));
#15832=DIRECTION('',(-3.69499511157397E-16,2.14359602894637E-16,-1.));
#15833=DIRECTION('center_axis',(0.487215765823115,-0.112342322983794,-0.866025403784439));
#15834=DIRECTION('ref_axis',(-0.843882460654216,0.194582611248245,-0.5));
#15835=DIRECTION('',(-0.843882460654216,0.194582611248245,-0.5));
#15836=DIRECTION('center_axis',(-0.487215765823116,0.112342322983932,0.86602540378442));
#15837=DIRECTION('ref_axis',(-0.616523841583692,-0.746591155021291,-0.250000000005721));
#15838=DIRECTION('',(-0.224684645967589,-0.974431531646231,-6.60780807231409E-17));
#15839=DIRECTION('',(-0.224684645967589,-0.974431531646231,-6.60780807231409E-17));
#15840=DIRECTION('center_axis',(-0.487215765823115,0.112342322983794,-0.866025403784439));
#15841=DIRECTION('ref_axis',(-0.843882460654216,0.194582611248245,0.5));
#15842=DIRECTION('',(-0.843882460654216,0.194582611248245,0.5));
#15843=DIRECTION('',(-0.224684645967589,-0.974431531646231,-6.60780807231409E-17));
#15844=DIRECTION('center_axis',(0.487215765823073,-0.11234232298389,0.86602540378445));
#15845=DIRECTION('ref_axis',(0.227358619055838,-0.941173766287018,-0.249999999988262));
#15846=DIRECTION('center_axis',(-0.974431531646231,0.224684645967589,4.0821528608577E-16));
#15847=DIRECTION('ref_axis',(3.69499511157397E-16,-2.14359602894637E-16,
1.));
#15848=DIRECTION('',(3.69499511157397E-16,-2.14359602894637E-16,1.));
#15849=DIRECTION('center_axis',(0.974431531646239,-0.224684645967554,2.62889778835188E-14));
#15850=DIRECTION('ref_axis',(0.194582611247985,0.843882460653167,-0.500000000001871));
#15851=DIRECTION('',(-0.224684645967589,-0.974431531646231,-6.60780807231409E-17));
#15852=DIRECTION('center_axis',(0.974431531646148,-0.224684645967948,8.109997424295E-14));
#15853=DIRECTION('ref_axis',(0.194582611256729,0.843882460689772,0.499999999936689));
#15854=DIRECTION('center_axis',(-0.487215765823115,0.112342322983794,0.866025403784439));
#15855=DIRECTION('ref_axis',(0.843882460654216,-0.194582611248245,0.5));
#15856=DIRECTION('',(0.843882460654216,-0.194582611248245,0.5));
#15857=DIRECTION('center_axis',(0.487215765823131,-0.112342322983759,-0.866025403784434));
#15858=DIRECTION('ref_axis',(-0.22735861905635,0.941173766286857,-0.249999999988406));
#15859=DIRECTION('',(-0.224684645967589,-0.974431531646231,-6.60780807231409E-17));
#15860=DIRECTION('center_axis',(0.487215765823115,-0.112342322983794,0.866025403784439));
#15861=DIRECTION('ref_axis',(0.843882460654216,-0.194582611248245,-0.5));
#15862=DIRECTION('',(-0.224684645967589,-0.974431531646231,-6.60780807231409E-17));
#15863=DIRECTION('center_axis',(-0.487215765823103,0.112342322983935,-0.866025403784427));
#15864=DIRECTION('ref_axis',(0.616523841604247,0.746591154999503,-0.250000000020098));
#15865=DIRECTION('',(0.843882460654216,-0.194582611248245,-0.5));
#15866=DIRECTION('center_axis',(0.974431531646231,-0.224684645967589,9.25562468266162E-17));
#15867=DIRECTION('ref_axis',(1.18468060663251E-16,1.01843928311571E-16,
-1.));
#15868=DIRECTION('center_axis',(-0.974431531646193,0.224684645967751,2.94355350819261E-14));
#15869=DIRECTION('ref_axis',(0.194582611249943,0.843882460661004,-0.499999999987883));
#15870=DIRECTION('',(1.18468060663251E-16,1.01843928311571E-16,-1.));
#15871=DIRECTION('center_axis',(-0.974431531646256,0.224684645967479,3.31911033510058E-14));
#15872=DIRECTION('ref_axis',(0.194582611244197,0.843882460637021,0.500000000030596));
#15873=DIRECTION('center_axis',(0.224684645967589,0.974431531646231,1.25857889322102E-16));
#15874=DIRECTION('ref_axis',(2.08745462991212E-17,1.24347063228184E-16,
-1.));
#15875=DIRECTION('center_axis',(0.224684645967592,0.97443153164623,4.52473261763703E-15));
#15876=DIRECTION('ref_axis',(0.843882460654121,-0.194582611248228,0.500000000000167));
#15877=DIRECTION('center_axis',(0.22468464596757,0.974431531646235,1.02704248305103E-14));
#15878=DIRECTION('ref_axis',(0.843882460654164,-0.19458261124821,-0.500000000000101));
#15879=DIRECTION('center_axis',(0.224684645967572,0.974431531646235,-8.04396909802231E-15));
#15880=DIRECTION('ref_axis',(0.843882460654151,-0.194582611248211,0.500000000000123));
#15881=DIRECTION('center_axis',(0.224684645967561,0.974431531646237,1.49387997534668E-14));
#15882=DIRECTION('ref_axis',(0.843882460654115,-0.194582611248188,-0.500000000000192));
#15883=DIRECTION('center_axis',(-0.185637535122341,0.768465162225134,0.612372435695795));
#15884=DIRECTION('ref_axis',(-0.843882460654216,0.194582611248245,-0.5));
#15885=DIRECTION('',(-0.785005807280206,-0.490824550811397,0.377964473009226));
#15886=DIRECTION('center_axis',(0.503389608706702,0.609589125432954,0.612372435695794));
#15887=DIRECTION('ref_axis',(-0.843882460654216,0.194582611248245,0.5));
#15888=DIRECTION('',(-0.490824550811399,0.785005807280205,-0.377964473009226));
#15889=DIRECTION('center_axis',(-0.530151107036863,0.847903180621225,2.35478172332082E-17));
#15890=DIRECTION('ref_axis',(1.18468060663251E-16,1.01843928311571E-16,
-1.));
#15891=DIRECTION('',(0.785005807280206,0.490824550811397,-0.377964473009226));
#15892=DIRECTION('',(-0.785005807280206,-0.490824550811397,-0.377964473009227));
#15893=DIRECTION('center_axis',(0.847903180621223,0.530151107036865,-1.99656829969769E-16));
#15894=DIRECTION('ref_axis',(3.69499511157397E-16,-2.14359602894637E-16,
1.));
#15895=DIRECTION('',(-0.4908245508114,0.785005807280206,0.377964473009223));
#15896=DIRECTION('',(0.490824550811399,-0.785005807280205,0.377964473009226));
#15897=DIRECTION('center_axis',(-0.185637535122341,0.768465162225134,-0.612372435695794));
#15898=DIRECTION('ref_axis',(0.843882460654216,-0.194582611248245,-0.5));
#15899=DIRECTION('',(0.785005807280206,0.490824550811397,0.377964473009226));
#15900=DIRECTION('center_axis',(0.503389608706703,0.609589125432952,-0.612372435695796));
#15901=DIRECTION('ref_axis',(0.843882460654216,-0.194582611248245,0.5));
#15902=DIRECTION('',(0.4908245508114,-0.785005807280206,-0.377964473009223));
#15903=DIRECTION('center_axis',(0.4908245508114,-0.785005807280206,-0.377964473009223));
#15904=DIRECTION('ref_axis',(-0.847903180621223,-0.530151107036865,-2.77555756156289E-17));
#15905=DIRECTION('center_axis',(9.16975147669649E-9,5.73796578879224E-9,
1.));
#15906=DIRECTION('ref_axis',(0.530161597891661,-0.847896621128402,3.75170931248065E-12));
#15907=DIRECTION('center_axis',(0.490824550811399,-0.785005807280205,0.377964473009226));
#15908=DIRECTION('ref_axis',(-0.847903180621223,-0.530151107036865,5.55111512312578E-17));
#15909=DIRECTION('center_axis',(0.785005807280206,0.490824550811397,0.377964473009227));
#15910=DIRECTION('ref_axis',(0.530151107036863,-0.847903180621225,-2.77555756156289E-16));
#15911=DIRECTION('center_axis',(-2.08293517271166E-9,3.33669624293654E-9,
1.));
#15912=DIRECTION('ref_axis',(0.847906432817937,0.530145905563706,-2.8017192176462E-12));
#15913=DIRECTION('center_axis',(0.785005807280206,0.490824550811397,-0.377964473009226));
#15914=DIRECTION('ref_axis',(0.530151107036863,-0.847903180621224,3.05311331771918E-16));
#15915=DIRECTION('center_axis',(-0.974431531646231,0.224684645967589,-1.26428912495664E-17));
#15916=DIRECTION('ref_axis',(0.224684645967589,0.974431531646231,1.23259516440783E-32));
#15917=DIRECTION('',(-0.974431531646231,0.224684645967589,-1.26428912495664E-17));
#15918=DIRECTION('',(0.974431531646231,-0.224684645967589,1.26428912495664E-17));
#15919=DIRECTION('center_axis',(-0.974431531646231,0.224684645967589,-1.26428912495664E-17));
#15920=DIRECTION('ref_axis',(0.224684645967589,0.974431531646231,1.23259516440783E-32));
#15921=DIRECTION('',(0.974431531646231,-0.224684645967589,1.26428912495664E-17));
#15922=DIRECTION('',(-0.974431531646231,0.224684645967589,-1.26428912495664E-17));
#15923=DIRECTION('center_axis',(0.224684645967589,0.974431531646231,1.25857889322102E-16));
#15924=DIRECTION('ref_axis',(2.08745462991212E-17,1.24347063228184E-16,
-1.));
#15925=DIRECTION('center_axis',(-0.974431531646231,0.224684645967589,7.59805975586106E-18));
#15926=DIRECTION('ref_axis',(-2.08745462991212E-17,-1.24347063228184E-16,
1.));
#15927=DIRECTION('center_axis',(-0.974431531646231,0.224684645967589,-1.26428912495664E-17));
#15928=DIRECTION('ref_axis',(0.224684645967589,0.974431531646231,1.42518815884655E-32));
#15929=DIRECTION('center_axis',(0.974431531646231,-0.224684645967589,1.26428912495664E-17));
#15930=DIRECTION('ref_axis',(1.23196318847518E-17,-2.84066354441556E-18,
-1.));
#15931=DIRECTION('center_axis',(0.0216454139389726,-0.98876345800245,-0.147913150782639));
#15932=DIRECTION('ref_axis',(-0.999760469446545,-0.021886153888323,1.85181731060524E-16));
#15933=DIRECTION('center_axis',(-0.843042330772965,-0.426528196188075,0.327648174695716));
#15934=DIRECTION('ref_axis',(-0.451448225784322,0.892297315605168,-2.31759056390501E-15));
#15935=DIRECTION('center_axis',(-0.974431531646231,0.224684645967589,-1.26428912495664E-17));
#15936=DIRECTION('ref_axis',(0.224684645967589,0.974431531646231,1.42518815884655E-32));
#15937=DIRECTION('center_axis',(-2.08745462991212E-17,-1.24347063228184E-16,
1.));
#15938=DIRECTION('ref_axis',(-0.974431531646231,0.224684645967589,7.59805975586112E-18));
#15939=DIRECTION('center_axis',(-0.974431531646231,0.224684645967589,-1.26428912495664E-17));
#15940=DIRECTION('ref_axis',(0.224684645967589,0.974431531646231,1.42518815884655E-32));
#15941=DIRECTION('center_axis',(0.974431531646231,-0.224684645967589,1.26428912495664E-17));
#15942=DIRECTION('ref_axis',(1.23196318847518E-17,-2.84066354441556E-18,
-1.));
#15943=DIRECTION('center_axis',(-2.08745462991212E-17,-1.24347063228184E-16,
1.));
#15944=DIRECTION('ref_axis',(0.974431531646231,-0.224684645967589,-7.59805975586112E-18));
#15945=DIRECTION('center_axis',(-2.08745462991212E-17,-1.24347063228184E-16,
1.));
#15946=DIRECTION('ref_axis',(0.974431531646231,-0.224684645967589,-7.59805975586112E-18));
#15947=DIRECTION('center_axis',(-0.974431531646231,0.224684645967589,-1.26428912495664E-17));
#15948=DIRECTION('ref_axis',(0.224684645967589,0.974431531646231,1.42518815884655E-32));
#15949=DIRECTION('center_axis',(0.843042330772967,0.426528196188067,0.327648174695721));
#15950=DIRECTION('ref_axis',(-0.451448225784312,0.892297315605173,-3.66373598126302E-15));
#15951=DIRECTION('center_axis',(0.021645413938973,-0.98876345800245,0.14791315078264));
#15952=DIRECTION('ref_axis',(-0.999760469446545,-0.0218861538883235,-1.16226472890446E-16));
#15953=DIRECTION('center_axis',(0.224684645967589,0.974431531646231,-2.56661170621381E-16));
#15954=DIRECTION('ref_axis',(-5.76678242546919E-17,-2.50098737602707E-16,
-1.));
#15955=DIRECTION('center_axis',(0.19458261124829,0.843882460654178,0.500000000000046));
#15956=DIRECTION('ref_axis',(-0.112342322997118,-0.48721576582009,0.866025403784412));
#15957=DIRECTION('center_axis',(-0.19458261124826,-0.843882460654214,0.499999999999998));
#15958=DIRECTION('ref_axis',(-0.11234232298209,-0.487215765823506,-0.86602540378444));
#15959=DIRECTION('center_axis',(0.112342322983794,0.487215765823116,-0.866025403784439));
#15960=DIRECTION('ref_axis',(-0.194582611248246,-0.843882460654216,-0.5));
#15961=DIRECTION('center_axis',(0.,0.,1.));
#15962=DIRECTION('ref_axis',(-0.224684645969392,-0.974431531645815,0.));
#15963=DIRECTION('center_axis',(0.112342322983794,0.487215765823116,0.866025403784439));
#15964=DIRECTION('ref_axis',(0.194582611248243,0.843882460654216,-0.5));
#15965=DIRECTION('center_axis',(0.,0.,1.));
#15966=DIRECTION('ref_axis',(-0.224684645964876,-0.974431531646856,0.));
#15967=DIRECTION('center_axis',(-0.112342322983794,-0.487215765823116,-0.866025403784439));
#15968=DIRECTION('ref_axis',(-0.194582611248246,-0.843882460654216,0.5));
#15969=DIRECTION('center_axis',(0.194582611248052,0.843882460654175,0.500000000000144));
#15970=DIRECTION('ref_axis',(-0.112342322985073,-0.487215765822968,0.866025403784356));
#15971=DIRECTION('center_axis',(-0.112342322983794,-0.487215765823115,0.866025403784439));
#15972=DIRECTION('ref_axis',(0.194582611248243,0.843882460654217,0.5));
#15973=DIRECTION('center_axis',(-0.19458261124824,-0.843882460654216,0.500000000000002));
#15974=DIRECTION('ref_axis',(-0.112342322980795,-0.487215765823809,-0.866025403784437));
#15975=DIRECTION('center_axis',(-0.224684645967589,-0.974431531646231,9.52915449491202E-17));
#15976=DIRECTION('ref_axis',(2.14105470405976E-17,9.28550860977068E-17,
1.));
#15977=DIRECTION('center_axis',(2.08745462991212E-17,1.24347063228184E-16,
-1.));
#15978=DIRECTION('ref_axis',(-0.974431531646231,0.224684645967587,7.59805975586085E-18));
#19399=CARTESIAN_POINT('',(0.,0.,0.));
#19400=CARTESIAN_POINT('Origin',(290.197052756605,75.7062702018219,258.073593133703));
#19401=CARTESIAN_POINT('',(251.28301830691,84.6790771867611,258.573593133703));
#19402=CARTESIAN_POINT('',(251.850698433645,84.5481813729906,257.573593133703));
#19403=CARTESIAN_POINT('Ctrl Pts',(251.28301830691,84.6790771867611,258.573593133703));
#19404=CARTESIAN_POINT('Ctrl Pts',(251.268603243666,84.6165607113056,258.573593133703));
#19405=CARTESIAN_POINT('Ctrl Pts',(251.258879081903,84.5491576952367,258.560454544981));
#19406=CARTESIAN_POINT('Ctrl Pts',(251.253717921743,84.4239190897031,258.508711173615));
#19407=CARTESIAN_POINT('Ctrl Pts',(251.258359391243,84.3660629060774,258.4701484502));
#19408=CARTESIAN_POINT('Ctrl Pts',(251.279707190674,84.2692747335277,258.380631525734));
#19409=CARTESIAN_POINT('Ctrl Pts',(251.298791240693,84.2253450690978,258.322746863925));
#19410=CARTESIAN_POINT('Ctrl Pts',(251.350351032782,84.1622186524674,258.199249594304));
#19411=CARTESIAN_POINT('Ctrl Pts',(251.382858032475,84.1429364355382,258.133693745596));
#19412=CARTESIAN_POINT('Ctrl Pts',(251.451741110902,84.1270533595221,258.011254161343));
#19413=CARTESIAN_POINT('Ctrl Pts',(251.493650046494,84.1299802798894,257.945064916044));
#19414=CARTESIAN_POINT('Ctrl Pts',(251.581308030854,84.1614864113044,257.82231806015));
#19415=CARTESIAN_POINT('Ctrl Pts',(251.627007294045,84.1900499387627,257.765720879009));
#19416=CARTESIAN_POINT('Ctrl Pts',(251.706009704231,84.2617248254449,257.678127980836));
#19417=CARTESIAN_POINT('Ctrl Pts',(251.745188081272,84.3083492613558,257.639781389305));
#19418=CARTESIAN_POINT('Ctrl Pts',(251.810210027717,84.4193221435049,257.587468702232));
#19419=CARTESIAN_POINT('Ctrl Pts',(251.835859543139,84.4838268073212,257.573593133703));
#19420=CARTESIAN_POINT('Ctrl Pts',(251.850698433645,84.5481813729906,257.573593133703));
#19421=CARTESIAN_POINT('',(139.64640668573,110.42027268846,257.573593133703));
#19422=CARTESIAN_POINT('',(290.197052756605,75.7062702018219,257.573593133703));
#19423=CARTESIAN_POINT('Origin',(139.64640668573,110.42027268846,258.073593133703));
#19424=CARTESIAN_POINT('Ctrl Pts',(251.850698433645,84.5481813729906,257.573593133703));
#19425=CARTESIAN_POINT('Ctrl Pts',(251.864800464293,84.6093402619923,257.573593133703));
#19426=CARTESIAN_POINT('Ctrl Pts',(251.870281693377,84.6753901958754,257.586153033938));
#19427=CARTESIAN_POINT('Ctrl Pts',(251.86254067835,84.7986066327571,257.634024355935));
#19428=CARTESIAN_POINT('Ctrl Pts',(251.849537380392,84.8558232696689,257.669241832604));
#19429=CARTESIAN_POINT('Ctrl Pts',(251.812123690221,84.957939080529,257.754170475265));
#19430=CARTESIAN_POINT('Ctrl Pts',(251.782979802506,85.0070349671363,257.81235564874));
#19431=CARTESIAN_POINT('Ctrl Pts',(251.715900228166,85.0786514884424,257.93946956097));
#19432=CARTESIAN_POINT('Ctrl Pts',(251.678004374675,85.1011208931129,258.008448170203));
#19433=CARTESIAN_POINT('Ctrl Pts',(251.60659972071,85.1175853945944,258.135369851765));
#19434=CARTESIAN_POINT('Ctrl Pts',(251.567893496343,85.1140577619974,258.202697763481));
#19435=CARTESIAN_POINT('Ctrl Pts',(251.492031699182,85.0775518559062,258.329014288151));
#19436=CARTESIAN_POINT('Ctrl Pts',(251.4548040378,85.044514145115,258.387942404826));
#19437=CARTESIAN_POINT('Ctrl Pts',(251.393730641083,84.9644905748009,258.475703765116));
#19438=CARTESIAN_POINT('Ctrl Pts',(251.365353141457,84.9151907353916,258.512264506913));
#19439=CARTESIAN_POINT('Ctrl Pts',(251.31702147063,84.8027912190808,258.561229944453));
#19440=CARTESIAN_POINT('Ctrl Pts',(251.296997530561,84.7397034759105,258.573593133703));
#19441=CARTESIAN_POINT('Ctrl Pts',(251.28301830691,84.6790771867611,258.573593133703));
#19442=CARTESIAN_POINT('Origin',(277.041252647849,78.7397376070303,227.073593133703));
#19443=CARTESIAN_POINT('',(288.247215261781,76.155864178403,225.073593133703));
#19444=CARTESIAN_POINT('Origin',(277.041252647849,78.7397376070303,225.073593133703));
#19445=CARTESIAN_POINT('',(290.196078325073,75.7064948864679,227.073593133703));
#19446=CARTESIAN_POINT('Origin',(288.247215261781,76.155864178403,227.073593133703));
#19447=CARTESIAN_POINT('',(263.886426970625,81.7729803275927,227.073593133703));
#19448=CARTESIAN_POINT('Origin',(277.041252647849,78.7397376070303,227.073593133703));
#19449=CARTESIAN_POINT('Origin',(277.041252647849,78.7397376070303,227.073593133703));
#19450=CARTESIAN_POINT('Origin',(277.041252647849,78.7397376070303,279.073593133703));
#19451=CARTESIAN_POINT('',(263.886426970625,81.7729803275927,279.073593133703));
#19452=CARTESIAN_POINT('',(290.196078325073,75.7064948864678,279.073593133703));
#19453=CARTESIAN_POINT('Origin',(277.041252647849,78.7397376070303,279.073593133703));
#19454=CARTESIAN_POINT('Origin',(277.041252647849,78.7397376070303,279.073593133703));
#19455=CARTESIAN_POINT('',(288.247215261781,76.155864178403,281.073593133703));
#19456=CARTESIAN_POINT('Origin',(288.247215261781,76.155864178403,279.073593133703));
#19457=CARTESIAN_POINT('Origin',(277.041252647849,78.7397376070303,281.073593133703));
#19458=CARTESIAN_POINT('Origin',(139.64640668573,110.42027268846,253.073593133703));
#19459=CARTESIAN_POINT('',(139.64640668573,110.42027268846,245.573593133703));
#19460=CARTESIAN_POINT('Origin',(139.64640668573,110.42027268846,253.073593133703));
#19461=CARTESIAN_POINT('',(125.029933711037,113.790542377974,245.573593133703));
#19462=CARTESIAN_POINT('',(139.64640668573,110.42027268846,245.573593133703));
#19463=CARTESIAN_POINT('Origin',(125.029933711037,113.790542377974,253.073593133703));
#19464=CARTESIAN_POINT('Origin',(255.074370622327,80.7261481941816,260.573593133704));
#19465=CARTESIAN_POINT('',(255.074370622327,80.7261481941816,265.573593133704));
#19466=CARTESIAN_POINT('Origin',(255.074370622327,80.7261481941816,260.573593133704));
#19467=CARTESIAN_POINT('',(264.061756461031,119.703409460031,265.573593133704));
#19468=CARTESIAN_POINT('',(255.074370622327,80.7261481941816,265.573593133704));
#19469=CARTESIAN_POINT('Origin',(264.061756461031,119.703409460031,260.573593133704));
#19470=CARTESIAN_POINT('Origin',(239.288983046701,153.123984191655,281.073593133703));
#19471=CARTESIAN_POINT('',(243.430317056198,152.169074446293,269.073593133703));
#19472=CARTESIAN_POINT('Origin',(239.288983046701,153.123984191655,269.073593133703));
#19473=CARTESIAN_POINT('',(243.430317056198,152.169074446293,251.073593133703));
#19474=CARTESIAN_POINT('',(243.430317056198,152.169074446293,281.073593133703));
#19475=CARTESIAN_POINT('Origin',(239.288983046701,153.123984191655,251.073593133703));
#19476=CARTESIAN_POINT('Origin',(277.041252647849,78.7397376070303,281.073593133703));
#19477=CARTESIAN_POINT('',(284.836704901019,76.9422604392896,281.073593133703));
#19478=CARTESIAN_POINT('Origin',(277.041252647849,78.7397376070303,281.073593133703));
#19479=CARTESIAN_POINT('',(284.836704901019,76.9422604392896,225.073593133703));
#19480=CARTESIAN_POINT('',(284.836704901019,76.9422604392896,281.073593133703));
#19481=CARTESIAN_POINT('Origin',(277.041252647849,78.7397376070303,225.073593133703));
#19482=CARTESIAN_POINT('Origin',(261.812330085074,110.608660518952,263.143363115103));
#19483=CARTESIAN_POINT('',(260.506630277985,120.523151270375,266.635682465084));
#19484=CARTESIAN_POINT('',(267.32755142688,118.950381708081,266.635682465084));
#19485=CARTESIAN_POINT('Origin',(263.917090852633,119.73676648918,252.326565285529));
#19486=CARTESIAN_POINT('',(260.455987287139,120.461895956422,266.697317490661));
#19487=CARTESIAN_POINT('Origin',(262.326343033394,112.718291331958,260.527055021389));
#19488=CARTESIAN_POINT('',(260.359612810304,120.043930907366,267.192605719228));
#19489=CARTESIAN_POINT('',(261.400356029357,124.557514844643,261.84401258248));
#19490=CARTESIAN_POINT('',(263.599526276829,118.359525358802,269.233847171548));
#19491=CARTESIAN_POINT('Origin',(260.627227793702,105.469007847775,269.233847171476));
#19492=CARTESIAN_POINT('',(267.249884248594,118.455170539444,267.192605719228));
#19493=CARTESIAN_POINT('Origin',(260.62722779321,105.469007845778,269.23384717163));
#19494=CARTESIAN_POINT('',(267.346258725429,118.8731355885,266.697317490661));
#19495=CARTESIAN_POINT('',(266.846226172141,116.704551773281,269.267087472061));
#19496=CARTESIAN_POINT('Origin',(262.311555516519,112.776310611233,260.572594253834));
#19497=CARTESIAN_POINT('Origin',(261.395367346685,108.800340960407,255.860966009446));
#19498=CARTESIAN_POINT('',(263.599526276829,118.359525358802,251.913339095859));
#19499=CARTESIAN_POINT('',(267.249884248594,118.455170539444,253.954580548178));
#19500=CARTESIAN_POINT('Origin',(260.62722779329,105.469007845961,251.913339095793));
#19501=CARTESIAN_POINT('',(260.359612810304,120.043930907366,253.954580548178));
#19502=CARTESIAN_POINT('Origin',(260.627227793615,105.469007846882,251.913339095865));
#19503=CARTESIAN_POINT('',(260.455987287139,120.461895956422,254.449868776745));
#19504=CARTESIAN_POINT('',(260.983393290967,122.749195286098,257.160316542069));
#19505=CARTESIAN_POINT('',(260.506630277985,120.523151270375,254.511503802322));
#19506=CARTESIAN_POINT('Origin',(262.319364171497,112.747732317274,260.596894987617));
#19507=CARTESIAN_POINT('',(267.32755142688,118.950381708081,254.511503802323));
#19508=CARTESIAN_POINT('Origin',(263.917090852491,119.736766489213,268.820620983067));
#19509=CARTESIAN_POINT('',(267.346258725429,118.8731355885,254.449868776745));
#19510=CARTESIAN_POINT('Origin',(262.33579074407,112.805792616964,260.54516207062));
#19511=CARTESIAN_POINT('',(266.429263433752,114.896232214736,249.737241652488));
#19512=CARTESIAN_POINT('Origin',(260.546821162919,105.120293514534,260.573593133703));
#19513=CARTESIAN_POINT('',(265.60821119059,93.6908433533151,260.573593133703));
#19514=CARTESIAN_POINT('Origin',(258.299974703243,95.375978198072,260.573593133703));
#19515=CARTESIAN_POINT('',(267.855057650266,103.435158669777,260.573593133703));
#19516=CARTESIAN_POINT('',(267.855057650266,103.435158669777,260.573593133703));
#19517=CARTESIAN_POINT('',(264.200939406592,104.277726092156,267.068783662087));
#19518=CARTESIAN_POINT('Origin',(260.546821162919,105.120293514534,260.573593133703));
#19519=CARTESIAN_POINT('',(256.892702919245,105.962860936913,267.068783662087));
#19520=CARTESIAN_POINT('Origin',(260.546821162919,105.120293514534,260.573593133703));
#19521=CARTESIAN_POINT('',(253.238584675572,106.805428359291,260.573593133703));
#19522=CARTESIAN_POINT('Origin',(260.546821162919,105.120293514534,260.573593133703));
#19523=CARTESIAN_POINT('',(256.892702919245,105.962860936913,254.07840260532));
#19524=CARTESIAN_POINT('Origin',(260.546821162919,105.120293514534,260.573593133703));
#19525=CARTESIAN_POINT('',(264.200939406592,104.277726092156,254.07840260532));
#19526=CARTESIAN_POINT('Origin',(260.546821162919,105.120293514534,260.573593133703));
#19527=CARTESIAN_POINT('Origin',(260.546821162919,105.120293514534,260.573593133703));
#19528=CARTESIAN_POINT('Origin',(244.644544516272,152.915336968997,253.073593133703));
#19529=CARTESIAN_POINT('',(246.891390975948,162.65965228546,251.073593133703));
#19530=CARTESIAN_POINT('',(254.062847596205,149.554449125806,251.073593133703));
#19531=CARTESIAN_POINT('Origin',(244.644544516272,152.915336968997,251.073593133703));
#19532=CARTESIAN_POINT('',(246.891390975948,162.65965228546,269.073593133703));
#19533=CARTESIAN_POINT('',(246.891390975948,162.65965228546,251.073593133703));
#19534=CARTESIAN_POINT('',(254.062847596205,149.554449125806,269.073593133703));
#19535=CARTESIAN_POINT('Origin',(244.644544516272,152.915336968997,269.073593133703));
#19536=CARTESIAN_POINT('',(254.062847596205,149.554449125806,269.073593133703));
#19537=CARTESIAN_POINT('Origin',(131.363738666737,112.330092179185,253.073593133703));
#19538=CARTESIAN_POINT('',(126.195991809483,89.9181669513215,253.073593133703));
#19539=CARTESIAN_POINT('Origin',(131.363738666737,112.330092179185,253.073593133703));
#19540=CARTESIAN_POINT('',(131.068149467714,88.7947437214835,253.073593133703));
#19541=CARTESIAN_POINT('',(126.195991809483,89.9181669513215,253.073593133703));
#19542=CARTESIAN_POINT('Origin',(136.235896324969,111.206668949347,253.073593133703));
#19543=CARTESIAN_POINT('Origin',(131.363738666737,112.330092179185,253.073593133703));
#19544=CARTESIAN_POINT('',(130.95580714473,88.3075279556604,253.073593133703));
#19545=CARTESIAN_POINT('Origin',(136.235896324969,111.206668949347,253.073593133703));
#19546=CARTESIAN_POINT('',(131.930238676376,88.0828433096928,253.073593133703));
#19547=CARTESIAN_POINT('',(126.083649486499,89.4309511854984,253.073593133703));
#19548=CARTESIAN_POINT('Origin',(137.210327856615,110.981984303379,253.073593133703));
#19549=CARTESIAN_POINT('Origin',(131.363738666737,112.330092179185,253.073593133703));
#19550=CARTESIAN_POINT('',(131.593211707425,86.6211960122235,253.073593133703));
#19551=CARTESIAN_POINT('Origin',(137.210327856615,110.981984303379,253.073593133703));
#19552=CARTESIAN_POINT('',(209.547734239124,68.6464243348164,253.073593133703));
#19553=CARTESIAN_POINT('',(125.746622517548,87.969303888029,253.073593133703));
#19554=CARTESIAN_POINT('Origin',(215.164850388313,93.0072126259722,253.073593133703));
#19555=CARTESIAN_POINT('Origin',(131.363738666737,112.330092179185,253.073593133703));
#19556=CARTESIAN_POINT('',(209.098364947188,66.6975612715239,253.073593133703));
#19557=CARTESIAN_POINT('Origin',(215.164850388313,93.0072126259722,253.073593133703));
#19558=CARTESIAN_POINT('',(210.560012244658,66.3605343025725,253.073593133703));
#19559=CARTESIAN_POINT('',(125.297253225612,86.0204408247366,253.073593133703));
#19560=CARTESIAN_POINT('',(221.513065902147,113.862671378776,269.073593133703));
#19561=CARTESIAN_POINT('Origin',(216.626497685783,92.6701856570208,253.073593133703));
#19562=CARTESIAN_POINT('',(222.676316926623,118.907557612938,251.073593133703));
#19563=CARTESIAN_POINT('Origin',(216.626497685783,92.6701856570208,253.073593133703));
#19564=CARTESIAN_POINT('Origin',(216.626497685783,92.6701856570208,253.073593133703));
#19565=CARTESIAN_POINT('Origin',(216.626497685783,92.6701856570208,253.073593133703));
#19566=CARTESIAN_POINT('',(240.538123974849,111.65376571076,251.073593133703));
#19567=CARTESIAN_POINT('',(238.543161711281,106.063231272255,269.073593133703));
#19568=CARTESIAN_POINT('Origin',(232.30684086269,88.5870277819392,253.073593133703));
#19569=CARTESIAN_POINT('Ctrl Pts',(238.543161711281,106.063231272255,269.073593133703));
#19570=CARTESIAN_POINT('Ctrl Pts',(230.852920983076,109.661454372805,269.073593133703));
#19571=CARTESIAN_POINT('Ctrl Pts',(221.513065902155,113.862671378773,269.073593133703));
#19572=CARTESIAN_POINT('',(235.819539119684,64.6411442799677,253.073593133703));
#19573=CARTESIAN_POINT('',(210.560012244658,66.3605343025725,253.073593133703));
#19574=CARTESIAN_POINT('',(240.249036425902,83.8513659038506,275.837689461751));
#19575=CARTESIAN_POINT('Origin',(240.987285976938,87.0530695078311,253.073593133703));
#19576=CARTESIAN_POINT('',(243.448117813726,97.7254148544326,273.29846276181));
#19577=CARTESIAN_POINT('Origin',(240.987285976938,87.0530695078311,253.073593133703));
#19578=CARTESIAN_POINT('',(243.448117813726,97.7254148544326,232.848723505596));
#19579=CARTESIAN_POINT('Origin',(240.987285976938,87.0530695078311,253.073593133703));
#19580=CARTESIAN_POINT('',(240.249036425902,83.8513659038506,230.309496805655));
#19581=CARTESIAN_POINT('Origin',(240.987285976938,87.0530695078311,253.073593133703));
#19582=CARTESIAN_POINT('Origin',(240.987285976938,87.0530695078311,253.073593133703));
#19583=CARTESIAN_POINT('Ctrl Pts',(222.676316926623,118.907557612938,251.073593133703));
#19584=CARTESIAN_POINT('Ctrl Pts',(228.630385342599,116.489953848209,251.073593133703));
#19585=CARTESIAN_POINT('Ctrl Pts',(234.584338031647,114.07206503216,251.073593133703));
#19586=CARTESIAN_POINT('Ctrl Pts',(240.538123974849,111.65376571076,251.073593133703));
#19587=CARTESIAN_POINT('Origin',(277.041252647849,78.7397376070303,225.073593133703));
#19588=CARTESIAN_POINT('',(263.886426970625,81.7729803275927,278.073593133703));
#19589=CARTESIAN_POINT('',(263.886426970625,81.7729803275927,225.073593133703));
#19590=CARTESIAN_POINT('',(263.544486310321,78.4442745295379,277.78120466771));
#19591=CARTESIAN_POINT('Ctrl Pts',(263.886446492733,81.7729758257347,278.073577619317));
#19592=CARTESIAN_POINT('Ctrl Pts',(263.85275455139,81.6268667898238,278.073579192226));
#19593=CARTESIAN_POINT('Ctrl Pts',(263.821493169456,81.4802343246266,278.071810719886));
#19594=CARTESIAN_POINT('Ctrl Pts',(263.792761752791,81.333477957104,278.068267543646));
#19595=CARTESIAN_POINT('Ctrl Pts',(263.752444668704,81.1275434959372,278.063295615668));
#19596=CARTESIAN_POINT('Ctrl Pts',(263.716974024298,80.9209501746423,278.054856597271));
#19597=CARTESIAN_POINT('Ctrl Pts',(263.686312053167,80.7134721297003,278.042963391396));
#19598=CARTESIAN_POINT('Ctrl Pts',(263.669333854775,80.5985870365692,278.036377865371));
#19599=CARTESIAN_POINT('Ctrl Pts',(263.653830777329,80.4834305611799,278.028732724067));
#19600=CARTESIAN_POINT('Ctrl Pts',(263.639801959899,80.3679634694504,278.020026203797));
#19601=CARTESIAN_POINT('Ctrl Pts',(263.629457986628,80.2828252518821,278.013606559846));
#19602=CARTESIAN_POINT('Ctrl Pts',(263.619941007641,80.1977065301477,278.006621309609));
#19603=CARTESIAN_POINT('Ctrl Pts',(263.61124379958,80.1126083918287,277.999079084841));
#19604=CARTESIAN_POINT('Ctrl Pts',(263.590437455768,79.9090279886416,277.981035809284));
#19605=CARTESIAN_POINT('Ctrl Pts',(263.57432785594,79.7056452709986,277.959809986454));
#19606=CARTESIAN_POINT('Ctrl Pts',(263.562830679749,79.5024395682177,277.935503430205));
#19607=CARTESIAN_POINT('Ctrl Pts',(263.551203283478,79.2969323035088,277.910921571423));
#19608=CARTESIAN_POINT('Ctrl Pts',(263.544293467851,79.0916056610182,277.883188588102));
#19609=CARTESIAN_POINT('Ctrl Pts',(263.542058389097,78.8864524133771,277.852383645832));
#19610=CARTESIAN_POINT('Ctrl Pts',(263.540451601139,78.7389686760395,277.830238112839));
#19611=CARTESIAN_POINT('Ctrl Pts',(263.541261700963,78.5915748264037,277.806504400391));
#19612=CARTESIAN_POINT('Ctrl Pts',(263.544486310321,78.4442745295379,277.78120466771));
#19613=CARTESIAN_POINT('',(264.697446773203,73.2734363904916,272.907655056344));
#19614=CARTESIAN_POINT('Ctrl Pts',(263.544486310321,78.4442745295379,277.78120466771));
#19615=CARTESIAN_POINT('Ctrl Pts',(263.547122992337,78.3238307793806,277.760517709776));
#19616=CARTESIAN_POINT('Ctrl Pts',(263.551293306596,78.205570043004,277.73432802133));
#19617=CARTESIAN_POINT('Ctrl Pts',(263.556873433881,78.0893078590764,277.703178796516));
#19618=CARTESIAN_POINT('Ctrl Pts',(263.5624795862,77.9725034424917,277.671884295515));
#19619=CARTESIAN_POINT('Ctrl Pts',(263.569508560945,77.8577154073319,277.635584233554));
#19620=CARTESIAN_POINT('Ctrl Pts',(263.5778464509,77.7447342870386,277.594783472228));
#19621=CARTESIAN_POINT('Ctrl Pts',(263.582583675622,77.6805433515511,277.57160226256));
#19622=CARTESIAN_POINT('Ctrl Pts',(263.587743651842,77.6169353572849,277.546967348406));
#19623=CARTESIAN_POINT('Ctrl Pts',(263.593307356281,77.5538702101861,277.52096425551));
#19624=CARTESIAN_POINT('Ctrl Pts',(263.603116432212,77.4426833519792,277.475119564176));
#19625=CARTESIAN_POINT('Ctrl Pts',(263.614188157078,77.3331122049833,277.424934853952));
#19626=CARTESIAN_POINT('Ctrl Pts',(263.626398085071,77.2251933445278,277.370779250483));
#19627=CARTESIAN_POINT('Ctrl Pts',(263.639089736436,77.1130167163494,277.314487023449));
#19628=CARTESIAN_POINT('Ctrl Pts',(263.653011113268,77.0026258188698,277.253904489932));
#19629=CARTESIAN_POINT('Ctrl Pts',(263.668008001099,76.8940658959719,277.189500756005));
#19630=CARTESIAN_POINT('Ctrl Pts',(263.672343279029,76.8626835556453,277.170883020818));
#19631=CARTESIAN_POINT('Ctrl Pts',(263.676768348929,76.8314542219291,277.151946290177));
#19632=CARTESIAN_POINT('Ctrl Pts',(263.681279292772,76.8003789551962,277.132702662197));
#19633=CARTESIAN_POINT('Ctrl Pts',(263.684570894048,76.7777035703618,277.11866073381));
#19634=CARTESIAN_POINT('Ctrl Pts',(263.68790110023,76.755157409625,277.10448259259));
#19635=CARTESIAN_POINT('Ctrl Pts',(263.691268503701,76.732740170163,277.090171883745));
#19636=CARTESIAN_POINT('Ctrl Pts',(263.709908083934,76.6086540791465,277.010957851916));
#19637=CARTESIAN_POINT('Ctrl Pts',(263.729710767152,76.4883513320883,276.927778617926));
#19638=CARTESIAN_POINT('Ctrl Pts',(263.750512514209,76.3714290619651,276.841087289969));
#19639=CARTESIAN_POINT('Ctrl Pts',(263.771934050831,76.25102308431,276.751812987597));
#19640=CARTESIAN_POINT('Ctrl Pts',(263.794415147851,76.1342022342419,276.658813972525));
#19641=CARTESIAN_POINT('Ctrl Pts',(263.817791248369,76.0205596546528,276.562540155481));
#19642=CARTESIAN_POINT('Ctrl Pts',(263.842448812904,75.9006872560012,276.460988664675));
#19643=CARTESIAN_POINT('Ctrl Pts',(263.86810223401,75.7843512561059,276.355793378961));
#19644=CARTESIAN_POINT('Ctrl Pts',(263.894573572594,75.6711080942386,276.247435360569));
#19645=CARTESIAN_POINT('Ctrl Pts',(263.916073581254,75.5791320518042,276.159427029352));
#19646=CARTESIAN_POINT('Ctrl Pts',(263.938113471031,75.4891969946826,276.069331328785));
#19647=CARTESIAN_POINT('Ctrl Pts',(263.960604308298,75.4010793409905,275.977386216045));
#19648=CARTESIAN_POINT('Ctrl Pts',(263.966186804265,75.3792074808841,275.954564334628));
#19649=CARTESIAN_POINT('Ctrl Pts',(263.971800969941,75.3574410130864,275.931613553638));
#19650=CARTESIAN_POINT('Ctrl Pts',(263.977445212981,75.3357801371126,275.90853904003));
#19651=CARTESIAN_POINT('Ctrl Pts',(264.012422701034,75.2015472514492,275.765545813408));
#19652=CARTESIAN_POINT('Ctrl Pts',(264.048568414587,75.0713158394443,275.617760857594));
#19653=CARTESIAN_POINT('Ctrl Pts',(264.085470719744,74.9453104927299,275.466568118245));
#19654=CARTESIAN_POINT('Ctrl Pts',(264.100639812602,74.8935146280335,275.404418702568));
#19655=CARTESIAN_POINT('Ctrl Pts',(264.115936918988,74.8424326620172,275.341692923535));
#19656=CARTESIAN_POINT('Ctrl Pts',(264.131334181614,74.7920794157389,275.278484566265));
#19657=CARTESIAN_POINT('Ctrl Pts',(264.136682122934,74.7745901897056,275.256530366105));
#19658=CARTESIAN_POINT('Ctrl Pts',(264.142041182813,74.7571908096217,275.234521931448));
#19659=CARTESIAN_POINT('Ctrl Pts',(264.147410915155,74.7398797847651,275.212460526197));
#19660=CARTESIAN_POINT('Ctrl Pts',(264.191265460638,74.5985008335307,275.032285270083));
#19661=CARTESIAN_POINT('Ctrl Pts',(264.235856933395,74.4629273361703,274.848488464814));
#19662=CARTESIAN_POINT('Ctrl Pts',(264.280980144503,74.3323009810995,274.661588044547));
#19663=CARTESIAN_POINT('Ctrl Pts',(264.291813083473,74.3009409050408,274.616717992161));
#19664=CARTESIAN_POINT('Ctrl Pts',(264.302676726821,74.2698661512641,274.571668927922));
#19665=CARTESIAN_POINT('Ctrl Pts',(264.313568343616,74.2390651848461,274.526447774819));
#19666=CARTESIAN_POINT('Ctrl Pts',(264.317765143417,74.2271968376442,274.509022985654));
#19667=CARTESIAN_POINT('Ctrl Pts',(264.32196588765,74.2153690830843,274.491572522455));
#19668=CARTESIAN_POINT('Ctrl Pts',(264.326170501729,74.2035814297529,274.474096678514));
#19669=CARTESIAN_POINT('Ctrl Pts',(264.369955565245,74.0808298192456,274.29211066922));
#19670=CARTESIAN_POINT('Ctrl Pts',(264.414158406344,73.9624286077785,274.107379181318));
#19671=CARTESIAN_POINT('Ctrl Pts',(264.458698703332,73.8478348019593,273.920240767794));
#19672=CARTESIAN_POINT('Ctrl Pts',(264.475771742853,73.803909082825,273.848507489255));
#19673=CARTESIAN_POINT('Ctrl Pts',(264.492894372165,73.7605432081688,273.776420191835));
#19674=CARTESIAN_POINT('Ctrl Pts',(264.510062044817,73.7177081324413,273.703996648076));
#19675=CARTESIAN_POINT('Ctrl Pts',(264.541713431899,73.6387347276007,273.570472106702));
#19676=CARTESIAN_POINT('Ctrl Pts',(264.573627236761,73.5613001852101,273.435322169166));
#19677=CARTESIAN_POINT('Ctrl Pts',(264.605605641687,73.4856481451905,273.299400074616));
#19678=CARTESIAN_POINT('Ctrl Pts',(264.636222180717,73.4132179023013,273.169266500958));
#19679=CARTESIAN_POINT('Ctrl Pts',(264.66689779028,73.342420324327,273.038425986335));
#19680=CARTESIAN_POINT('Ctrl Pts',(264.697446430188,73.2734364754757,272.907654931384));
#19681=CARTESIAN_POINT('',(264.697446773204,73.273436390491,233.239531211061));
#19682=CARTESIAN_POINT('',(264.697446473732,73.2734363771458,281.073593133703));
#19683=CARTESIAN_POINT('',(263.544486310321,78.4442745295379,228.365981599697));
#19684=CARTESIAN_POINT('Ctrl Pts',(264.697446430188,73.2734364754763,233.239531336022));
#19685=CARTESIAN_POINT('Ctrl Pts',(264.663254910726,73.3506465449807,233.093166028613));
#19686=CARTESIAN_POINT('Ctrl Pts',(264.62902021271,73.4298652314763,232.947195179886));
#19687=CARTESIAN_POINT('Ctrl Pts',(264.594902967084,73.5110401054218,232.802302791382));
#19688=CARTESIAN_POINT('Ctrl Pts',(264.566508978667,73.5785976818973,232.681716480109));
#19689=CARTESIAN_POINT('Ctrl Pts',(264.538196350838,73.647509921883,232.561876938124));
#19690=CARTESIAN_POINT('Ctrl Pts',(264.510055257259,73.7177250681167,232.443160985242));
#19691=CARTESIAN_POINT('Ctrl Pts',(264.465269218582,73.8294711964643,232.254226705116));
#19692=CARTESIAN_POINT('Ctrl Pts',(264.420789806233,73.9448269326336,232.067578466915));
#19693=CARTESIAN_POINT('Ctrl Pts',(264.376697369361,74.0643200580235,231.883541793551));
#19694=CARTESIAN_POINT('Ctrl Pts',(264.35979481214,74.1101269930158,231.812992497049));
#19695=CARTESIAN_POINT('Ctrl Pts',(264.342949112854,74.1565423392094,231.742827319498));
#19696=CARTESIAN_POINT('Ctrl Pts',(264.326164814146,74.2035973749484,231.673065948251));
#19697=CARTESIAN_POINT('Ctrl Pts',(264.321962099464,74.2153797492373,231.655598007274));
#19698=CARTESIAN_POINT('Ctrl Pts',(264.317763251177,74.227202188807,231.638155424292));
#19699=CARTESIAN_POINT('Ctrl Pts',(264.313568343771,74.2390651844082,231.620738492203));
#19700=CARTESIAN_POINT('Ctrl Pts',(264.268201373635,74.3673607854903,231.432378330354));
#19701=CARTESIAN_POINT('Ctrl Pts',(264.223318747672,74.5004034612182,231.247001665634));
#19702=CARTESIAN_POINT('Ctrl Pts',(264.179122612568,74.6390415540256,231.065119437598));
#19703=CARTESIAN_POINT('Ctrl Pts',(264.168509912247,74.6723323503493,231.02144454215));
#19704=CARTESIAN_POINT('Ctrl Pts',(264.157936852948,74.705945969639,230.977971270434));
#19705=CARTESIAN_POINT('Ctrl Pts',(264.147406342131,74.7398945273785,230.934706951834));
#19706=CARTESIAN_POINT('Ctrl Pts',(264.142038140199,74.7572006881552,230.912651839528));
#19707=CARTESIAN_POINT('Ctrl Pts',(264.136680604834,74.774595154308,230.890649668241));
#19708=CARTESIAN_POINT('Ctrl Pts',(264.131334181738,74.7920794153349,230.868701700738));
#19709=CARTESIAN_POINT('Ctrl Pts',(264.093877580934,74.9145727110991,230.714936044264));
#19710=CARTESIAN_POINT('Ctrl Pts',(264.057012652599,75.0413796191397,230.56402291816));
#19711=CARTESIAN_POINT('Ctrl Pts',(264.021144891591,75.1722820846851,230.417326682335));
#19712=CARTESIAN_POINT('Ctrl Pts',(264.006398845075,75.2260990443088,230.357016547095));
#19713=CARTESIAN_POINT('Ctrl Pts',(263.991821517935,75.2806080558477,230.29741972076));
#19714=CARTESIAN_POINT('Ctrl Pts',(263.977441810656,75.3357931942203,230.238633316917));
#19715=CARTESIAN_POINT('Ctrl Pts',(263.971798713818,75.3574497602277,230.215563489193));
#19716=CARTESIAN_POINT('Ctrl Pts',(263.966185682656,75.3792118752832,230.192617345688));
#19717=CARTESIAN_POINT('Ctrl Pts',(263.960604308547,75.4010793400128,230.169800050216));
#19718=CARTESIAN_POINT('Ctrl Pts',(263.93293244652,75.5094959154173,230.05667431453));
#19719=CARTESIAN_POINT('Ctrl Pts',(263.905942876101,75.6206628873982,229.946347126665));
#19720=CARTESIAN_POINT('Ctrl Pts',(263.879802393058,75.7349992059669,229.839265251712));
#19721=CARTESIAN_POINT('Ctrl Pts',(263.854558246421,75.8454150229674,229.735855129217));
#19722=CARTESIAN_POINT('Ctrl Pts',(263.830105880425,75.9587863617574,229.63547133516));
#19723=CARTESIAN_POINT('Ctrl Pts',(263.806607422103,76.0755167676874,229.538553045713));
#19724=CARTESIAN_POINT('Ctrl Pts',(263.784247108639,76.1865933511585,229.446328981367));
#19725=CARTESIAN_POINT('Ctrl Pts',(263.762750505002,76.3007113943396,229.357242760094));
#19726=CARTESIAN_POINT('Ctrl Pts',(263.742268982999,76.41824476033,229.271708885874));
#19727=CARTESIAN_POINT('Ctrl Pts',(263.724465455108,76.5204104372433,229.197358712329));
#19728=CARTESIAN_POINT('Ctrl Pts',(263.707429038303,76.6251569658246,229.1256930543));
#19729=CARTESIAN_POINT('Ctrl Pts',(263.691267273814,76.7327483577029,229.057009150204));
#19730=CARTESIAN_POINT('Ctrl Pts',(263.687900289533,76.7551628982351,229.042700215954));
#19731=CARTESIAN_POINT('Ctrl Pts',(263.684570493643,76.7777063287377,229.028523817602));
#19732=CARTESIAN_POINT('Ctrl Pts',(263.681279293248,76.8003789519183,229.014483599006));
#19733=CARTESIAN_POINT('Ctrl Pts',(263.665616777329,76.9082758524226,228.94766750733));
#19734=CARTESIAN_POINT('Ctrl Pts',(263.650990460361,77.0180303308622,228.88455500451));
#19735=CARTESIAN_POINT('Ctrl Pts',(263.637560028327,77.1295969108204,228.825635123568));
#19736=CARTESIAN_POINT('Ctrl Pts',(263.624663225137,77.2367306367194,228.769056295237));
#19737=CARTESIAN_POINT('Ctrl Pts',(263.612869251473,77.345534854029,228.716343689266));
#19738=CARTESIAN_POINT('Ctrl Pts',(263.602307206215,77.4559709595898,228.667883260715));
#19739=CARTESIAN_POINT('Ctrl Pts',(263.599199542263,77.4884645056732,228.653624779213));
#19740=CARTESIAN_POINT('Ctrl Pts',(263.596198439943,77.5210993620194,228.639734085692));
#19741=CARTESIAN_POINT('Ctrl Pts',(263.593306963389,77.5538746636589,228.626220175638));
#19742=CARTESIAN_POINT('Ctrl Pts',(263.583514536842,77.6648732237023,228.58045325721));
#19743=CARTESIAN_POINT('Ctrl Pts',(263.5749720485,77.7775539423449,228.538921908102));
#19744=CARTESIAN_POINT('Ctrl Pts',(263.567786046187,77.8921334806293,228.502103165652));
#19745=CARTESIAN_POINT('Ctrl Pts',(263.560624490531,78.0063232212909,228.465409679932));
#19746=CARTESIAN_POINT('Ctrl Pts',(263.554810288292,78.1223996733709,228.433397020835));
#19747=CARTESIAN_POINT('Ctrl Pts',(263.550461447433,78.2405621917892,228.406585073276));
#19748=CARTESIAN_POINT('Ctrl Pts',(263.547987548257,78.3077805992609,228.391332720497));
#19749=CARTESIAN_POINT('Ctrl Pts',(263.545988077553,78.3756737364794,228.377764209574));
#19750=CARTESIAN_POINT('Ctrl Pts',(263.544486310321,78.4442745295379,228.365981599697));
#19751=CARTESIAN_POINT('',(263.886426970624,81.772980327589,228.073593133703));
#19752=CARTESIAN_POINT('Ctrl Pts',(263.544486310321,78.4442745295379,228.365981599697));
#19753=CARTESIAN_POINT('Ctrl Pts',(263.532233262231,79.0039943036223,228.269846283192));
#19754=CARTESIAN_POINT('Ctrl Pts',(263.554916335949,79.564270344569,228.1964953478));
#19755=CARTESIAN_POINT('Ctrl Pts',(263.668901959567,80.6739967475123,228.098538799407));
#19756=CARTESIAN_POINT('Ctrl Pts',(263.760142632711,81.2252996425734,228.073593133703));
#19757=CARTESIAN_POINT('Ctrl Pts',(263.886426970624,81.772980327589,228.073593133703));
#19758=CARTESIAN_POINT('',(263.886426970625,81.7729803275927,225.073593133703));
#19759=CARTESIAN_POINT('',(270.946701599761,90.7857513677001,231.090039190109));
#19760=CARTESIAN_POINT('Ctrl Pts',(263.886426970624,81.772980327589,228.073593133703));
#19761=CARTESIAN_POINT('Ctrl Pts',(264.001135944375,82.2704599862669,228.073593133703));
#19762=CARTESIAN_POINT('Ctrl Pts',(264.146335943853,82.7685441967117,228.094687286035));
#19763=CARTESIAN_POINT('Ctrl Pts',(264.487097581211,83.7300632379758,228.176938403303));
#19764=CARTESIAN_POINT('Ctrl Pts',(264.682739293133,84.1958745673196,228.237768468517));
#19765=CARTESIAN_POINT('Ctrl Pts',(265.122345133427,85.0991343182584,228.395675688844));
#19766=CARTESIAN_POINT('Ctrl Pts',(265.366315246832,85.5365782245936,228.492763582321));
#19767=CARTESIAN_POINT('Ctrl Pts',(265.902443031719,86.3835668852031,228.720687561053));
#19768=CARTESIAN_POINT('Ctrl Pts',(266.192653439003,86.7895749064117,228.850739559984));
#19769=CARTESIAN_POINT('Ctrl Pts',(266.807294497184,87.5577921493384,229.134683190109));
#19770=CARTESIAN_POINT('Ctrl Pts',(267.132911069831,87.9218946153554,229.289088480638));
#19771=CARTESIAN_POINT('Ctrl Pts',(267.820387108045,88.6120665546024,229.618387505555));
#19772=CARTESIAN_POINT('Ctrl Pts',(268.180775004094,88.9363519636559,229.792575966063));
#19773=CARTESIAN_POINT('Ctrl Pts',(269.297122750516,89.8390387465664,230.329375212186));
#19774=CARTESIAN_POINT('Ctrl Pts',(270.092871176763,90.3537650523302,230.709036602005));
#19775=CARTESIAN_POINT('Ctrl Pts',(270.946701599761,90.7857513677001,231.090039190109));
#19776=CARTESIAN_POINT('',(274.135356630693,91.9232791773928,234.607407821084));
#19777=CARTESIAN_POINT('Ctrl Pts',(274.135356630693,91.9232791773928,234.607407821084));
#19778=CARTESIAN_POINT('Ctrl Pts',(274.135356630693,91.9232791773928,234.535038320367));
#19779=CARTESIAN_POINT('Ctrl Pts',(274.131436756292,91.9224288106584,234.463064877428));
#19780=CARTESIAN_POINT('Ctrl Pts',(274.123796303849,91.920744045495,234.391656669208));
#19781=CARTESIAN_POINT('Ctrl Pts',(274.115830884442,91.9189876231853,234.317211296794));
#19782=CARTESIAN_POINT('Ctrl Pts',(274.103821772655,91.9163242964729,234.243380425369));
#19783=CARTESIAN_POINT('Ctrl Pts',(274.088051837444,91.9127833752737,234.170349753486));
#19784=CARTESIAN_POINT('Ctrl Pts',(274.073492261134,91.9095142234529,234.102924261494));
#19785=CARTESIAN_POINT('Ctrl Pts',(274.055727958994,91.9054971820186,234.036180864883));
#19786=CARTESIAN_POINT('Ctrl Pts',(274.035019617716,91.9007632709779,233.970259652222));
#19787=CARTESIAN_POINT('Ctrl Pts',(274.030590092907,91.8997506849808,233.956159071058));
#19788=CARTESIAN_POINT('Ctrl Pts',(274.026022031944,91.8987044218231,233.942084342085));
#19789=CARTESIAN_POINT('Ctrl Pts',(274.021317425863,91.8976246431716,233.928036589951));
#19790=CARTESIAN_POINT('Ctrl Pts',(273.996549383788,91.8919400008002,233.854080277806));
#19791=CARTESIAN_POINT('Ctrl Pts',(273.968405853511,91.8854043574047,233.781795504628));
#19792=CARTESIAN_POINT('Ctrl Pts',(273.937311798586,91.8780563768258,233.711117184978));
#19793=CARTESIAN_POINT('Ctrl Pts',(273.905247128146,91.8704790255848,233.638232608412));
#19794=CARTESIAN_POINT('Ctrl Pts',(273.870044967459,91.8620378190554,233.567056334283));
#19795=CARTESIAN_POINT('Ctrl Pts',(273.832220155868,91.852783418526,233.497490874661));
#19796=CARTESIAN_POINT('Ctrl Pts',(273.811999181047,91.8478360574629,233.460301491602));
#19797=CARTESIAN_POINT('Ctrl Pts',(273.791029483462,91.842656431848,233.423572028953));
#19798=CARTESIAN_POINT('Ctrl Pts',(273.769394948025,91.8372532137308,233.387284706976));
#19799=CARTESIAN_POINT('Ctrl Pts',(273.75731872463,91.8342371809058,233.367029416177));
#19800=CARTESIAN_POINT('Ctrl Pts',(273.745028222076,91.8311496969879,233.346904585884));
#19801=CARTESIAN_POINT('Ctrl Pts',(273.732538525545,91.8279922984367,233.326908576382));
#19802=CARTESIAN_POINT('Ctrl Pts',(273.689569052797,91.8171296044821,233.258114432083));
#19803=CARTESIAN_POINT('Ctrl Pts',(273.64403282093,91.8053830652006,233.190632216215));
#19804=CARTESIAN_POINT('Ctrl Pts',(273.596418421607,91.792813601476,233.124621978395));
#19805=CARTESIAN_POINT('Ctrl Pts',(273.545891715675,91.7794753339275,233.054574263372));
#19806=CARTESIAN_POINT('Ctrl Pts',(273.493025268019,91.7652103828472,232.986184379854));
#19807=CARTESIAN_POINT('Ctrl Pts',(273.43845586753,91.750105172685,232.919622166538));
#19808=CARTESIAN_POINT('Ctrl Pts',(273.424728915839,91.7463054518098,232.902878418605));
#19809=CARTESIAN_POINT('Ctrl Pts',(273.410894432972,91.7424526253429,232.886250209042));
#19810=CARTESIAN_POINT('Ctrl Pts',(273.396962980695,91.7385481935867,232.869740012722));
#19811=CARTESIAN_POINT('Ctrl Pts',(273.379603236693,91.733682948068,232.849166939948));
#19812=CARTESIAN_POINT('Ctrl Pts',(273.36208638432,91.7287357448304,232.828771019452));
#19813=CARTESIAN_POINT('Ctrl Pts',(273.344430059197,91.723708600085,232.80855424713));
#19814=CARTESIAN_POINT('Ctrl Pts',(273.261137520052,91.6999933791896,232.713182968666));
#19815=CARTESIAN_POINT('Ctrl Pts',(273.174290846884,91.6743883805731,232.62123981037));
#19816=CARTESIAN_POINT('Ctrl Pts',(273.084583825663,91.6468908813567,232.532417612095));
#19817=CARTESIAN_POINT('Ctrl Pts',(273.043592822645,91.6343260892366,232.491830922805));
#19818=CARTESIAN_POINT('Ctrl Pts',(273.002005218492,91.6213661190327,232.451895635956));
#19819=CARTESIAN_POINT('Ctrl Pts',(272.959890653297,91.6080105790183,232.412581106915));
#19820=CARTESIAN_POINT('Ctrl Pts',(272.940882337097,91.6019825854623,232.394836580863));
#19821=CARTESIAN_POINT('Ctrl Pts',(272.921780141506,91.5958782675561,232.377232616759));
#19822=CARTESIAN_POINT('Ctrl Pts',(272.902591220157,91.5896979801168,232.359766120084));
#19823=CARTESIAN_POINT('Ctrl Pts',(272.770031813146,91.5470038013668,232.239105432614));
#19824=CARTESIAN_POINT('Ctrl Pts',(272.634389128362,91.5010339939522,232.125630805735));
#19825=CARTESIAN_POINT('Ctrl Pts',(272.496134800693,91.4515980170925,232.018444263631));
#19826=CARTESIAN_POINT('Ctrl Pts',(272.361709975531,91.4035313658842,231.914226678366));
#19827=CARTESIAN_POINT('Ctrl Pts',(272.224816181694,91.3521879483791,231.815953774217));
#19828=CARTESIAN_POINT('Ctrl Pts',(272.085906933541,91.2973816581163,231.722756196414));
#19829=CARTESIAN_POINT('Ctrl Pts',(272.053657844897,91.2846578622823,231.70111950204));
#19830=CARTESIAN_POINT('Ctrl Pts',(272.021300214268,91.271747374894,231.679756161252));
#19831=CARTESIAN_POINT('Ctrl Pts',(271.988839875611,91.2586477742405,231.658654931275));
#19832=CARTESIAN_POINT('Ctrl Pts',(271.975359761063,91.2532077780899,231.649892022169));
#19833=CARTESIAN_POINT('Ctrl Pts',(271.961862581456,91.2477354286293,231.641175220404));
#19834=CARTESIAN_POINT('Ctrl Pts',(271.948348777553,91.2422305660915,231.632503737925));
#19835=CARTESIAN_POINT('Ctrl Pts',(271.75944749256,91.1652814247133,231.511290333106));
#19836=CARTESIAN_POINT('Ctrl Pts',(271.567168706644,91.0819855798593,231.399173785266));
#19837=CARTESIAN_POINT('Ctrl Pts',(271.371685966445,90.991522850765,231.296407213572));
#19838=CARTESIAN_POINT('Ctrl Pts',(271.231645955151,90.9267171211585,231.222787251798));
#19839=CARTESIAN_POINT('Ctrl Pts',(271.089961938186,90.8582323944569,231.153965888954));
#19840=CARTESIAN_POINT('Ctrl Pts',(270.946701599761,90.7857513677001,231.090039190109));
#19841=CARTESIAN_POINT('',(274.135356630693,91.9232791773928,271.539778446323));
#19842=CARTESIAN_POINT('',(274.135356630693,91.9232791773928,225.073593133703));
#19843=CARTESIAN_POINT('',(270.946701599761,90.7857513677001,275.057147077298));
#19844=CARTESIAN_POINT('Ctrl Pts',(270.946701599761,90.7857513677001,275.057147077298));
#19845=CARTESIAN_POINT('Ctrl Pts',(271.147148719625,90.8871654312007,274.967702065628));
#19846=CARTESIAN_POINT('Ctrl Pts',(271.34476324736,90.9808826077627,274.868561523026));
#19847=CARTESIAN_POINT('Ctrl Pts',(271.539328407034,91.0677140898358,274.759933194106));
#19848=CARTESIAN_POINT('Ctrl Pts',(271.67685557422,91.1290903802882,274.683149938679));
#19849=CARTESIAN_POINT('Ctrl Pts',(271.81285958917,91.1870253136085,274.601626202326));
#19850=CARTESIAN_POINT('Ctrl Pts',(271.947269297188,91.2417907833522,274.515433600296));
#19851=CARTESIAN_POINT('Ctrl Pts',(271.961599095474,91.2476294846334,274.506244363752));
#19852=CARTESIAN_POINT('Ctrl Pts',(271.975910489673,91.2534319294108,274.497001196149));
#19853=CARTESIAN_POINT('Ctrl Pts',(271.990203132732,91.2591983338119,274.487703508352));
#19854=CARTESIAN_POINT('Ctrl Pts',(272.098285900434,91.3028046104674,274.417393221716));
#19855=CARTESIAN_POINT('Ctrl Pts',(272.205337551487,91.3443656947214,274.343942722402));
#19856=CARTESIAN_POINT('Ctrl Pts',(272.311082571951,91.3839252173294,274.267188431155));
#19857=CARTESIAN_POINT('Ctrl Pts',(272.35211269782,91.3992747078759,274.23740699826));
#19858=CARTESIAN_POINT('Ctrl Pts',(272.392946253339,91.4143230179486,274.207128671626));
#19859=CARTESIAN_POINT('Ctrl Pts',(272.433567745757,91.4290732808565,274.176345871292));
#19860=CARTESIAN_POINT('Ctrl Pts',(272.451959857466,91.435751727831,274.162408404479));
#19861=CARTESIAN_POINT('Ctrl Pts',(272.470318707282,91.4423720860675,274.14835848214));
#19862=CARTESIAN_POINT('Ctrl Pts',(272.488636890527,91.4489329051577,274.134198442038));
#19863=CARTESIAN_POINT('Ctrl Pts',(272.577176988614,91.4806443231537,274.06575653801));
#19864=CARTESIAN_POINT('Ctrl Pts',(272.664928571698,91.5110220617877,273.994616949445));
#19865=CARTESIAN_POINT('Ctrl Pts',(272.751028463175,91.539884748222,273.921056877197));
#19866=CARTESIAN_POINT('Ctrl Pts',(272.803061616885,91.5573274717141,273.876601971615));
#19867=CARTESIAN_POINT('Ctrl Pts',(272.854492132878,91.5742172229607,273.831263556676));
#19868=CARTESIAN_POINT('Ctrl Pts',(272.905137133368,91.590517678791,273.785106949247));
#19869=CARTESIAN_POINT('Ctrl Pts',(272.925013081086,91.596914894799,273.766992499505));
#19870=CARTESIAN_POINT('Ctrl Pts',(272.944773927187,91.6032238307619,273.748751578454));
#19871=CARTESIAN_POINT('Ctrl Pts',(272.964413382458,91.609444741243,273.730379919488));
#19872=CARTESIAN_POINT('Ctrl Pts',(273.034955955629,91.6317895072633,273.664391118936));
#19873=CARTESIAN_POINT('Ctrl Pts',(273.104021449973,91.6530265267405,273.596655216366));
#19874=CARTESIAN_POINT('Ctrl Pts',(273.171289389613,91.6731554332118,273.526995740641));
#19875=CARTESIAN_POINT('Ctrl Pts',(273.230376538101,91.6908363625213,273.465807902753));
#19876=CARTESIAN_POINT('Ctrl Pts',(273.288076906538,91.7076624974713,273.403136222412));
#19877=CARTESIAN_POINT('Ctrl Pts',(273.344191153207,91.7236405759986,273.338888375723));
#19878=CARTESIAN_POINT('Ctrl Pts',(273.36228644354,91.7287930637726,273.318170224663));
#19879=CARTESIAN_POINT('Ctrl Pts',(273.380235891361,91.7338618607828,273.297266495054));
#19880=CARTESIAN_POINT('Ctrl Pts',(273.398019690814,91.7388444962522,273.276177765194));
#19881=CARTESIAN_POINT('Ctrl Pts',(273.453966754319,91.7545196518199,273.209833533649));
#19882=CARTESIAN_POINT('Ctrl Pts',(273.508419834158,91.7693827426634,273.141518011198));
#19883=CARTESIAN_POINT('Ctrl Pts',(273.560758070633,91.7833496634919,273.071236177951));
#19884=CARTESIAN_POINT('Ctrl Pts',(273.610309195982,91.7965728190913,273.004696986654));
#19885=CARTESIAN_POINT('Ctrl Pts',(273.657964349937,91.8089927169614,272.936395433542));
#19886=CARTESIAN_POINT('Ctrl Pts',(273.70323469989,91.8205482289851,272.866362499145));
#19887=CARTESIAN_POINT('Ctrl Pts',(273.712961851203,91.8230311391919,272.851314659874));
#19888=CARTESIAN_POINT('Ctrl Pts',(273.722579057508,91.8254741813287,272.836186985488));
#19889=CARTESIAN_POINT('Ctrl Pts',(273.732081738571,91.8278768144873,272.820979949206));
#19890=CARTESIAN_POINT('Ctrl Pts',(273.744956668504,91.8311320782775,272.800376340041));
#19891=CARTESIAN_POINT('Ctrl Pts',(273.757607589668,91.8343101457514,272.779659819711));
#19892=CARTESIAN_POINT('Ctrl Pts',(273.770020895007,91.8374100213599,272.758824248661));
#19893=CARTESIAN_POINT('Ctrl Pts',(273.832725777213,91.8530688108257,272.653574922014));
#19894=CARTESIAN_POINT('Ctrl Pts',(273.88937815834,91.8667377350326,272.545434259877));
#19895=CARTESIAN_POINT('Ctrl Pts',(273.938616077441,91.8783669180643,272.433109113283));
#19896=CARTESIAN_POINT('Ctrl Pts',(273.969165785573,91.8855822544134,272.363416882029));
#19897=CARTESIAN_POINT('Ctrl Pts',(273.996862422025,91.8920119710173,272.292114942464));
#19898=CARTESIAN_POINT('Ctrl Pts',(274.021380084588,91.8976390244009,272.218897869882));
#19899=CARTESIAN_POINT('Ctrl Pts',(274.026196873887,91.8987445266264,272.204513496541));
#19900=CARTESIAN_POINT('Ctrl Pts',(274.030872599235,91.8998153772765,272.190089704733));
#19901=CARTESIAN_POINT('Ctrl Pts',(274.035405043613,91.9008513765542,272.175627657681));
#19902=CARTESIAN_POINT('Ctrl Pts',(274.055251319512,91.9053877206955,272.112302495372));
#19903=CARTESIAN_POINT('Ctrl Pts',(274.072276528136,91.9092391436709,272.048499558861));
#19904=CARTESIAN_POINT('Ctrl Pts',(274.08637809056,91.9124075875364,271.984215131047));
#19905=CARTESIAN_POINT('Ctrl Pts',(274.100128678601,91.9154971718687,271.921530681072));
#19906=CARTESIAN_POINT('Ctrl Pts',(274.111099813145,91.9179373759246,271.858387904451));
#19907=CARTESIAN_POINT('Ctrl Pts',(274.119153279711,91.9197187509681,271.794763406625));
#19908=CARTESIAN_POINT('Ctrl Pts',(274.126895998593,91.9214313906211,271.733593896994));
#19909=CARTESIAN_POINT('Ctrl Pts',(274.131942127975,91.922535058773,271.6719787108));
#19910=CARTESIAN_POINT('Ctrl Pts',(274.134123443669,91.923010727664,271.609884997458));
#19911=CARTESIAN_POINT('Ctrl Pts',(274.134941983491,91.9231892226569,271.586584299993));
#19912=CARTESIAN_POINT('Ctrl Pts',(274.135356629434,91.9232791771153,271.563216125089));
#19913=CARTESIAN_POINT('Ctrl Pts',(274.135356630693,91.9232791773928,271.539778446323));
#19914=CARTESIAN_POINT('Ctrl Pts',(270.946701599761,90.7857513677001,275.057147077298));
#19915=CARTESIAN_POINT('Ctrl Pts',(270.092103000801,90.3533764019677,275.438492446616));
#19916=CARTESIAN_POINT('Ctrl Pts',(269.294515045443,89.8375330431696,275.819048322909));
#19917=CARTESIAN_POINT('Ctrl Pts',(268.174370042181,88.9308682907682,276.357698561063));
#19918=CARTESIAN_POINT('Ctrl Pts',(267.812566862767,88.6046709104441,276.532563521238));
#19919=CARTESIAN_POINT('Ctrl Pts',(267.128003174131,87.9165036644382,276.860429416162));
#19920=CARTESIAN_POINT('Ctrl Pts',(266.803853181977,87.5536763209671,277.014109934142));
#19921=CARTESIAN_POINT('Ctrl Pts',(266.192094255626,86.7886894429728,277.296687835193));
#19922=CARTESIAN_POINT('Ctrl Pts',(265.904476993744,86.3865438599545,277.425604060267));
#19923=CARTESIAN_POINT('Ctrl Pts',(265.502051757571,85.7511352760914,277.596731851499));
#19924=CARTESIAN_POINT('Ctrl Pts',(265.372514445692,85.533418720424,277.650143627071));
#19925=CARTESIAN_POINT('Ctrl Pts',(265.12700712324,85.0930287132427,277.747519903133));
#19926=CARTESIAN_POINT('Ctrl Pts',(265.010589450995,84.8697087087132,277.791682801321));
#19927=CARTESIAN_POINT('Ctrl Pts',(264.68025597584,84.1903680227695,277.910250222304));
#19928=CARTESIAN_POINT('Ctrl Pts',(264.485195531666,83.7249952768337,277.970754033365));
#19929=CARTESIAN_POINT('Ctrl Pts',(264.146458099391,82.7685882982612,278.052422184988));
#19930=CARTESIAN_POINT('Ctrl Pts',(264.002516023709,82.2764452320033,278.073593133703));
#19931=CARTESIAN_POINT('Ctrl Pts',(263.886426970625,81.7729803275927,278.073593133703));
#19932=CARTESIAN_POINT('Origin',(292.894242939747,87.3992238969307,278.073593133703));
#19933=CARTESIAN_POINT('',(243.683501728549,98.7462478875858,234.607407821084));
#19934=CARTESIAN_POINT('',(243.683501728549,98.7462478875858,271.539778446323));
#19935=CARTESIAN_POINT('',(243.683501728549,98.7462478875858,278.073593133703));
#19936=CARTESIAN_POINT('',(273.255484225105,91.9275333837837,271.539778446323));
#19937=CARTESIAN_POINT('',(273.710942204595,91.8225137784534,271.539778446323));
#19938=CARTESIAN_POINT('',(273.255484225105,91.9275333837837,234.607407821084));
#19939=CARTESIAN_POINT('',(273.255484225105,91.9275333837837,233.452176263355));
#19940=CARTESIAN_POINT('',(243.683501728549,98.7462478875858,234.607407821084));
#19941=CARTESIAN_POINT('Origin',(257.611187373776,70.1353745599898,281.073593133703));
#19942=CARTESIAN_POINT('',(259.352493380025,77.6872189302482,273.85820282453));
#19943=CARTESIAN_POINT('',(259.352493380025,77.6872189302482,232.288983442877));
#19944=CARTESIAN_POINT('',(259.352493380025,77.6872189302482,281.073593133703));
#19945=CARTESIAN_POINT('Ctrl Pts',(259.352493380025,77.6872189302482,232.288983442877));
#19946=CARTESIAN_POINT('Ctrl Pts',(259.799729931322,77.5840950237155,232.288983442877));
#19947=CARTESIAN_POINT('Ctrl Pts',(260.231148369232,77.4433515176037,232.295963080489));
#19948=CARTESIAN_POINT('Ctrl Pts',(260.647156973428,77.2660829175506,232.311173103591));
#19949=CARTESIAN_POINT('Ctrl Pts',(260.786178632926,77.2068433376293,232.316255985606));
#19950=CARTESIAN_POINT('Ctrl Pts',(260.92347921877,77.1435243769817,232.322258048075));
#19951=CARTESIAN_POINT('Ctrl Pts',(261.059073483003,77.0761656990271,232.329226123689));
#19952=CARTESIAN_POINT('Ctrl Pts',(261.060375152847,77.0755190731517,232.329293015412));
#19953=CARTESIAN_POINT('Ctrl Pts',(261.061676665124,77.07487207515,232.329359996202));
#19954=CARTESIAN_POINT('Ctrl Pts',(261.062978019842,77.0742247050601,232.3294270661));
#19955=CARTESIAN_POINT('Ctrl Pts',(261.33228449996,76.9402558817594,232.343306723991));
#19956=CARTESIAN_POINT('Ctrl Pts',(261.596147266426,76.789265470937,232.361264709447));
#19957=CARTESIAN_POINT('Ctrl Pts',(261.849676263299,76.623649486148,232.384109654213));
#19958=CARTESIAN_POINT('Ctrl Pts',(261.851636577294,76.622368925199,232.38428629383));
#19959=CARTESIAN_POINT('Ctrl Pts',(261.8535962632,76.6210874966772,232.384463224748));
#19960=CARTESIAN_POINT('Ctrl Pts',(261.855555318817,76.619805201697,232.384640447333));
#19961=CARTESIAN_POINT('Ctrl Pts',(262.108186840548,76.4544458676261,232.407494321975));
#19962=CARTESIAN_POINT('Ctrl Pts',(262.348506811958,76.2761308640001,232.434981980953));
#19963=CARTESIAN_POINT('Ctrl Pts',(262.576984544395,76.0854467300596,232.468251468614));
#19964=CARTESIAN_POINT('Ctrl Pts',(262.579684340403,76.0831935202688,232.468644595896));
#19965=CARTESIAN_POINT('Ctrl Pts',(262.582382478871,76.0809385862697,232.469038530122));
#19966=CARTESIAN_POINT('Ctrl Pts',(262.58507896041,76.0786819291588,232.469433273148));
#19967=CARTESIAN_POINT('Ctrl Pts',(262.812349292638,75.8884817723865,232.502703806442));
#19968=CARTESIAN_POINT('Ctrl Pts',(263.027844148003,75.6860350266864,232.541716928009));
#19969=CARTESIAN_POINT('Ctrl Pts',(263.231485141018,75.4715486344357,232.588031737839));
#19970=CARTESIAN_POINT('Ctrl Pts',(263.23511017773,75.4677305375262,232.588856193089));
#19971=CARTESIAN_POINT('Ctrl Pts',(263.238731445518,75.4639086400978,232.589682957477));
#19972=CARTESIAN_POINT('Ctrl Pts',(263.242348944987,75.460082942514,232.590512039929));
#19973=CARTESIAN_POINT('Ctrl Pts',(263.403005120879,75.2901805142746,232.627332284797));
#19974=CARTESIAN_POINT('Ctrl Pts',(263.55696374067,75.1117051982107,232.669024678028));
#19975=CARTESIAN_POINT('Ctrl Pts',(263.701646453658,74.9279097715543,232.715699089282));
#19976=CARTESIAN_POINT('Ctrl Pts',(263.738889682465,74.8805984170229,232.727713695187));
#19977=CARTESIAN_POINT('Ctrl Pts',(263.775518302732,74.8329342760175,232.740058480346));
#19978=CARTESIAN_POINT('Ctrl Pts',(263.811488351603,74.7849723248566,232.752735451858));
#19979=CARTESIAN_POINT('Ctrl Pts',(263.816088319008,74.7788387937955,232.754356624405));
#19980=CARTESIAN_POINT('Ctrl Pts',(263.820677519938,74.7727003868462,232.755983225899));
#19981=CARTESIAN_POINT('Ctrl Pts',(263.82525585932,74.7665572228774,232.757615259359));
#19982=CARTESIAN_POINT('Ctrl Pts',(263.987229223509,74.5492231958706,232.815353650487));
#19983=CARTESIAN_POINT('Ctrl Pts',(264.136085850256,74.3259353125209,232.879765865605));
#19984=CARTESIAN_POINT('Ctrl Pts',(264.272124827383,74.09724671866,232.952014823533));
#19985=CARTESIAN_POINT('Ctrl Pts',(264.405225297936,73.8734979071372,233.022703169626));
#19986=CARTESIAN_POINT('Ctrl Pts',(264.526056135609,73.6445794265254,233.10089378503));
#19987=CARTESIAN_POINT('Ctrl Pts',(264.634929493928,73.4110199756965,233.187638901472));
#19988=CARTESIAN_POINT('Ctrl Pts',(264.656225433704,73.3653350801831,233.20460649395));
#19989=CARTESIAN_POINT('Ctrl Pts',(264.67706396797,73.3194726457758,233.221901259064));
#19990=CARTESIAN_POINT('Ctrl Pts',(264.697447567359,73.2734366659659,233.239530880404));
#19991=CARTESIAN_POINT('Ctrl Pts',(264.697447567358,73.2734366659668,272.907655386999));
#19992=CARTESIAN_POINT('Ctrl Pts',(264.593340011719,73.5085616425729,272.997697226476));
#19993=CARTESIAN_POINT('Ctrl Pts',(264.477362758326,73.739158912752,273.079000675102));
#19994=CARTESIAN_POINT('Ctrl Pts',(264.349198619934,73.9646996202116,273.152606789554));
#19995=CARTESIAN_POINT('Ctrl Pts',(264.218208011609,74.1952142933692,273.227836177661));
#19996=CARTESIAN_POINT('Ctrl Pts',(264.074486792083,74.420446661668,273.295025414564));
#19997=CARTESIAN_POINT('Ctrl Pts',(263.917729942372,74.6398427726569,273.355326969753));
#19998=CARTESIAN_POINT('Ctrl Pts',(263.887394022256,74.6823007763035,273.366996655412));
#19999=CARTESIAN_POINT('Ctrl Pts',(263.856570013268,74.7245402454938,273.378408500692));
#20000=CARTESIAN_POINT('Ctrl Pts',(263.82525585932,74.7665572228779,273.389571008044));
#20001=CARTESIAN_POINT('Ctrl Pts',(263.820677519938,74.7727003868467,273.391203041504));
#20002=CARTESIAN_POINT('Ctrl Pts',(263.816088319007,74.778838793796,273.392829642998));
#20003=CARTESIAN_POINT('Ctrl Pts',(263.811488351602,74.7849723248571,273.394450815546));
#20004=CARTESIAN_POINT('Ctrl Pts',(263.671751693772,74.9712951953743,273.443698389183));
#20005=CARTESIAN_POINT('Ctrl Pts',(263.522076037587,75.1531271579415,273.487933669545));
#20006=CARTESIAN_POINT('Ctrl Pts',(263.365038680784,75.3272284309448,273.527269693373));
#20007=CARTESIAN_POINT('Ctrl Pts',(263.324615206953,75.3720443804524,273.537395301459));
#20008=CARTESIAN_POINT('Ctrl Pts',(263.283703950786,75.4163478301469,273.547196213751));
#20009=CARTESIAN_POINT('Ctrl Pts',(263.242348944987,75.4600829425142,273.556674227475));
#20010=CARTESIAN_POINT('Ctrl Pts',(263.238731445518,75.4639086400981,273.557503309927));
#20011=CARTESIAN_POINT('Ctrl Pts',(263.23511017773,75.4677305375265,273.558330074314));
#20012=CARTESIAN_POINT('Ctrl Pts',(263.231485141018,75.471548634436,273.559154529565));
#20013=CARTESIAN_POINT('Ctrl Pts',(263.027844148002,75.6860350266869,273.605469339391));
#20014=CARTESIAN_POINT('Ctrl Pts',(262.812349292638,75.8884817723866,273.644482460965));
#20015=CARTESIAN_POINT('Ctrl Pts',(262.58507896041,76.0786819291588,273.677752994258));
#20016=CARTESIAN_POINT('Ctrl Pts',(262.582382478871,76.0809385862696,273.678147737285));
#20017=CARTESIAN_POINT('Ctrl Pts',(262.579684340403,76.0831935202688,273.678541671511));
#20018=CARTESIAN_POINT('Ctrl Pts',(262.576984544395,76.0854467300596,273.678934798793));
#20019=CARTESIAN_POINT('Ctrl Pts',(262.348506811958,76.2761308640001,273.712204286454));
#20020=CARTESIAN_POINT('Ctrl Pts',(262.108186840548,76.4544458676262,273.739691945435));
#20021=CARTESIAN_POINT('Ctrl Pts',(261.855555318817,76.6198052016969,273.762545820075));
#20022=CARTESIAN_POINT('Ctrl Pts',(261.853596263201,76.6210874966771,273.762723042661));
#20023=CARTESIAN_POINT('Ctrl Pts',(261.851636577294,76.6223689251989,273.762899973578));
#20024=CARTESIAN_POINT('Ctrl Pts',(261.849676263299,76.6236494861479,273.763076613196));
#20025=CARTESIAN_POINT('Ctrl Pts',(261.596147266426,76.789265470937,273.785921557959));
#20026=CARTESIAN_POINT('Ctrl Pts',(261.33228449996,76.9402558817594,273.803879543416));
#20027=CARTESIAN_POINT('Ctrl Pts',(261.062978019842,77.0742247050601,273.817759201306));
#20028=CARTESIAN_POINT('Ctrl Pts',(261.061676665124,77.07487207515,273.817826271204));
#20029=CARTESIAN_POINT('Ctrl Pts',(261.060375152847,77.0755190731518,273.817893251995));
#20030=CARTESIAN_POINT('Ctrl Pts',(261.059073483003,77.0761656990271,273.817960143717));
#20031=CARTESIAN_POINT('Ctrl Pts',(260.65332096387,77.2777299275741,273.838811425665));
#20032=CARTESIAN_POINT('Ctrl Pts',(260.23229067611,77.4431241300129,273.85101306254));
#20033=CARTESIAN_POINT('Ctrl Pts',(259.795580893516,77.5712698272539,273.855817711116));
#20034=CARTESIAN_POINT('Ctrl Pts',(259.649641401155,77.614093502722,273.857423326566));
#20035=CARTESIAN_POINT('Ctrl Pts',(259.501950724621,77.6527570214662,273.85820282453));
#20036=CARTESIAN_POINT('Ctrl Pts',(259.352493380025,77.6872189302482,273.85820282453));
#20037=CARTESIAN_POINT('Origin',(239.8638627471,82.1809118495999,281.073593133703));
#20038=CARTESIAN_POINT('',(239.8638627471,82.1809118495999,273.85820282453));
#20039=CARTESIAN_POINT('',(239.8638627471,82.1809118495999,232.288983442877));
#20040=CARTESIAN_POINT('',(239.8638627471,82.1809118495999,281.073593133703));
#20041=CARTESIAN_POINT('',(259.352493380025,77.6872189302482,232.288983442877));
#20042=CARTESIAN_POINT('',(239.8638627471,82.1809118495999,273.85820282453));
#20043=CARTESIAN_POINT('Origin',(277.041252647849,78.7397376070303,225.073593133703));
#20044=CARTESIAN_POINT('Origin',(277.041252647849,78.7397376070303,281.073593133703));
#20045=CARTESIAN_POINT('Origin',(240.987285976938,87.0530695078311,253.073593133703));
#20046=CARTESIAN_POINT('Origin',(240.313232039036,84.1297749128924,232.288983442877));
#20047=CARTESIAN_POINT('Origin',(240.313232039036,84.1297749128924,273.85820282453));
#20048=CARTESIAN_POINT('Origin',(240.987285976938,87.0530695078311,253.073593133703));
#20049=CARTESIAN_POINT('Origin',(243.234132436614,96.7973848242934,234.607407821084));
#20050=CARTESIAN_POINT('Origin',(243.234132436614,96.7973848242934,271.539778446323));
#20051=CARTESIAN_POINT('Origin',(221.231335829438,119.31686398042,253.073593133703));
#20052=CARTESIAN_POINT('Origin',(142.827444005805,135.342772594535,253.073593133703));
#20053=CARTESIAN_POINT('Origin',(141.515985505207,134.105809943033,253.073593133703));
#20054=CARTESIAN_POINT('Origin',(136.531485523992,134.742017407048,253.073593133703));
#20055=CARTESIAN_POINT('',(133.779098610889,122.805231144382,271.693139315069));
#20056=CARTESIAN_POINT('',(136.194458555041,133.280370109579,253.073593133703));
#20057=CARTESIAN_POINT('',(133.779098610889,122.805231144382,271.693139315069));
#20058=CARTESIAN_POINT('',(128.948378722586,101.854953213988,271.693139315069));
#20059=CARTESIAN_POINT('',(128.948378722586,101.854953213988,271.693139315069));
#20060=CARTESIAN_POINT('',(126.533018778434,91.3798142487909,253.073593133703));
#20061=CARTESIAN_POINT('',(126.533018778434,91.3798142487909,253.073593133703));
#20062=CARTESIAN_POINT('',(128.948378722586,101.854953213988,234.454046952338));
#20063=CARTESIAN_POINT('',(128.948378722586,101.854953213988,234.454046952338));
#20064=CARTESIAN_POINT('',(133.779098610889,122.805231144382,234.454046952338));
#20065=CARTESIAN_POINT('',(133.779098610889,122.805231144382,234.454046952338));
#20066=CARTESIAN_POINT('',(136.194458555041,133.280370109579,253.073593133703));
#20067=CARTESIAN_POINT('Origin',(127.445293655188,124.265681343171,271.693139315069));
#20068=CARTESIAN_POINT('',(130.835085130986,134.516135662401,253.073593133703));
#20069=CARTESIAN_POINT('',(129.86065359934,134.740820308368,253.073593133703));
#20070=CARTESIAN_POINT('',(128.419725186835,124.040996697204,271.693139315069));
#20071=CARTESIAN_POINT('',(128.419725186835,124.040996697204,271.693139315069));
#20072=CARTESIAN_POINT('',(127.445293655188,124.265681343171,271.693139315069));
#20073=CARTESIAN_POINT('Origin',(129.86065359934,134.740820308368,253.073593133703));
#20074=CARTESIAN_POINT('',(128.419725186835,124.040996697204,234.454046952338));
#20075=CARTESIAN_POINT('',(127.445293655188,124.265681343171,234.454046952338));
#20076=CARTESIAN_POINT('',(130.835085130986,134.516135662401,253.073593133703));
#20077=CARTESIAN_POINT('Origin',(127.445293655188,124.265681343171,234.454046952338));
#20078=CARTESIAN_POINT('',(123.589005298532,103.09071876681,234.454046952338));
#20079=CARTESIAN_POINT('',(122.614573766885,103.315403412777,234.454046952338));
#20080=CARTESIAN_POINT('',(128.419725186835,124.040996697204,234.454046952338));
#20081=CARTESIAN_POINT('Origin',(122.614573766885,103.315403412777,234.454046952338));
#20082=CARTESIAN_POINT('',(121.17364535438,92.6155798016126,253.073593133703));
#20083=CARTESIAN_POINT('',(120.199213822734,92.8402644475802,253.073593133703));
#20084=CARTESIAN_POINT('',(123.589005298532,103.09071876681,234.454046952338));
#20085=CARTESIAN_POINT('Origin',(120.199213822734,92.8402644475802,253.073593133703));
#20086=CARTESIAN_POINT('',(123.589005298532,103.09071876681,271.693139315069));
#20087=CARTESIAN_POINT('',(122.614573766885,103.315403412777,271.693139315069));
#20088=CARTESIAN_POINT('',(121.17364535438,92.6155798016126,253.073593133703));
#20089=CARTESIAN_POINT('Origin',(122.614573766885,103.315403412777,271.693139315069));
#20090=CARTESIAN_POINT('',(123.589005298532,103.09071876681,271.693139315069));
#20091=CARTESIAN_POINT('Origin',(125.029933711037,113.790542377974,253.073593133703));
#20092=CARTESIAN_POINT('',(120.458657304398,93.9654410617858,253.073593133703));
#20093=CARTESIAN_POINT('',(122.744295507717,103.87799171988,270.693139315069));
#20094=CARTESIAN_POINT('',(122.809156378134,104.159285873431,271.193139315069));
#20095=CARTESIAN_POINT('',(127.315571914356,123.703093036068,270.693139315069));
#20096=CARTESIAN_POINT('',(127.445293655188,124.265681343171,270.693139315069));
#20097=CARTESIAN_POINT('',(129.601210117676,133.615643694162,253.073593133703));
#20098=CARTESIAN_POINT('',(129.666070988092,133.896937847714,252.573593133703));
#20099=CARTESIAN_POINT('',(127.315571914356,123.703093036068,235.454046952338));
#20100=CARTESIAN_POINT('',(127.25071104394,123.421798882517,234.954046952338));
#20101=CARTESIAN_POINT('',(122.744295507717,103.87799171988,235.454046952338));
#20102=CARTESIAN_POINT('',(122.614573766885,103.315403412777,235.454046952338));
#20103=CARTESIAN_POINT('',(120.393796433982,93.6841469082344,253.573593133703));
#20104=CARTESIAN_POINT('Origin',(257.838634424508,160.135434381298,253.073593133703));
#20105=CARTESIAN_POINT('',(237.375572259937,164.853811946618,253.073593133703));
#20106=CARTESIAN_POINT('',(233.477846133352,165.752550530488,253.073593133703));
#20107=CARTESIAN_POINT('',(233.477846133352,165.752550530488,253.073593133703));
#20108=CARTESIAN_POINT('',(237.375572259937,164.853811946618,265.706741519111));
#20109=CARTESIAN_POINT('',(237.375572259937,164.853811946618,265.706741519111));
#20110=CARTESIAN_POINT('',(233.477846133352,165.752550530488,265.706741519111));
#20111=CARTESIAN_POINT('',(233.477846133352,165.752550530488,265.706741519111));
#20112=CARTESIAN_POINT('',(233.477846133352,165.752550530488,269.073593133703));
#20113=CARTESIAN_POINT('',(233.477846133352,165.752550530488,265.706741519111));
#20114=CARTESIAN_POINT('',(233.477846133352,165.752550530488,269.073593133703));
#20115=CARTESIAN_POINT('',(233.477846133352,165.752550530488,251.073593133703));
#20116=CARTESIAN_POINT('',(246.891390975948,162.65965228546,251.073593133703));
#20117=CARTESIAN_POINT('',(233.477846133352,165.752550530488,251.073593133703));
#20118=CARTESIAN_POINT('Origin',(216.626497685783,92.6701856570208,253.073593133703));
#20119=CARTESIAN_POINT('',(219.996767375296,107.286658631714,269.073593133703));
#20120=CARTESIAN_POINT('',(234.488927040206,170.137492422896,265.706741519111));
#20121=CARTESIAN_POINT('',(234.488927040206,170.137492422896,265.706741519111));
#20122=CARTESIAN_POINT('',(234.488927040206,170.137492422896,253.073593133703));
#20123=CARTESIAN_POINT('',(234.488927040206,170.137492422896,265.706741519111));
#20124=CARTESIAN_POINT('',(234.488927040206,170.137492422896,253.073593133703));
#20125=CARTESIAN_POINT('',(219.996767375296,107.286658631714,251.073593133703));
#20126=CARTESIAN_POINT('Origin',(240.987285976938,87.0530695078311,251.073593133703));
#20127=CARTESIAN_POINT('',(237.536534944929,103.242335004298,251.073593133703));
#20128=CARTESIAN_POINT('Origin',(240.987285976938,87.0530695078311,269.073593133703));
#20129=CARTESIAN_POINT('',(237.536534944929,103.242335004298,269.073593133703));
#20130=CARTESIAN_POINT('Origin',(232.801789355145,89.9740347659234,253.073593133703));
#20131=CARTESIAN_POINT('Origin',(234.488927040206,170.137492422896,265.706741519111));
#20132=CARTESIAN_POINT('',(237.712599228888,166.315459244087,265.706741519111));
#20133=CARTESIAN_POINT('',(238.386653166791,169.238753839026,265.706741519111));
#20134=CARTESIAN_POINT('',(235.463358571852,169.912807776929,265.706741519111));
#20135=CARTESIAN_POINT('Origin',(234.789304633949,166.98951318199,265.706741519111));
#20136=CARTESIAN_POINT('',(234.488927040206,170.137492422896,265.706741519111));
#20137=CARTESIAN_POINT('Origin',(238.386653166791,169.238753839026,265.706741519111));
#20138=CARTESIAN_POINT('',(237.712599228888,166.315459244087,253.073593133703));
#20139=CARTESIAN_POINT('',(238.386653166791,169.238753839026,253.073593133703));
#20140=CARTESIAN_POINT('',(237.712599228888,166.315459244087,265.706741519111));
#20141=CARTESIAN_POINT('Origin',(234.488927040206,170.137492422896,253.073593133703));
#20142=CARTESIAN_POINT('',(235.463358571852,169.912807776929,253.073593133703));
#20143=CARTESIAN_POINT('',(234.488927040206,170.137492422896,253.073593133703));
#20144=CARTESIAN_POINT('Origin',(234.789304633949,166.98951318199,253.073593133703));
#20145=CARTESIAN_POINT('Origin',(258.849715331362,164.520376273706,253.073593133703));
#20146=CARTESIAN_POINT('',(235.463358571852,169.912807776929,253.073593133703));
#20147=CARTESIAN_POINT('Origin',(245.930348188225,108.490563204048,253.073593133703));
#20148=CARTESIAN_POINT('',(267.855057650266,103.435158669777,256.243466114781));
#20149=CARTESIAN_POINT('',(267.855057650266,103.435158669777,264.903720152625));
#20150=CARTESIAN_POINT('',(267.855057650266,103.435158669777,256.243466114781));
#20151=CARTESIAN_POINT('Origin',(245.930348188225,108.490563204048,253.073593133703));
#20152=CARTESIAN_POINT('',(260.546821162919,105.120293514534,251.913339095859));
#20153=CARTESIAN_POINT('',(267.855057650266,103.435158669777,256.243466114781));
#20154=CARTESIAN_POINT('',(260.546821162919,105.120293514534,251.913339095859));
#20155=CARTESIAN_POINT('Origin',(245.930348188225,108.490563204048,253.073593133703));
#20156=CARTESIAN_POINT('',(253.238584675572,106.805428359291,256.243466114781));
#20157=CARTESIAN_POINT('',(260.546821162919,105.120293514534,251.913339095859));
#20158=CARTESIAN_POINT('',(253.238584675572,106.805428359291,256.243466114781));
#20159=CARTESIAN_POINT('Origin',(245.930348188225,108.490563204048,253.073593133703));
#20160=CARTESIAN_POINT('',(253.238584675572,106.805428359291,264.903720152625));
#20161=CARTESIAN_POINT('',(253.238584675572,106.805428359291,256.243466114781));
#20162=CARTESIAN_POINT('',(253.238584675572,106.805428359291,264.903720152625));
#20163=CARTESIAN_POINT('Origin',(245.930348188225,108.490563204048,253.073593133703));
#20164=CARTESIAN_POINT('',(260.546821162919,105.120293514534,269.233847171548));
#20165=CARTESIAN_POINT('',(253.238584675572,106.805428359291,264.903720152625));
#20166=CARTESIAN_POINT('',(260.546821162919,105.120293514534,269.233847171548));
#20167=CARTESIAN_POINT('Origin',(245.930348188225,108.490563204048,253.073593133703));
#20168=CARTESIAN_POINT('',(267.855057650266,103.435158669777,264.903720152625));
#20169=CARTESIAN_POINT('',(260.546821162919,105.120293514534,269.233847171548));
#20170=CARTESIAN_POINT('',(267.855057650266,103.435158669777,264.903720152625));
#20171=CARTESIAN_POINT('Origin',(256.608854365086,121.421901333985,264.903720152625));
#20172=CARTESIAN_POINT('',(259.941647761247,120.140305384201,266.944961604945));
#20173=CARTESIAN_POINT('',(256.496512042102,120.934685568162,264.903720152625));
#20174=CARTESIAN_POINT('',(256.291289789483,120.044660203559,264.903720152625));
#20175=CARTESIAN_POINT('Origin',(253.318991306379,107.15414269192,264.903720152651));
#20176=CARTESIAN_POINT('',(256.608854365086,121.421901333985,264.903720152625));
#20177=CARTESIAN_POINT('',(263.917090852433,119.736766489228,269.233847171548));
#20178=CARTESIAN_POINT('Origin',(263.917090852433,119.736766489228,269.233847171548));
#20179=CARTESIAN_POINT('',(267.66784929765,118.358796062609,266.944961604945));
#20180=CARTESIAN_POINT('',(263.804748529449,119.249550723405,269.233847171548));
#20181=CARTESIAN_POINT('',(270.907762764176,116.674390514045,264.903720152625));
#20182=CARTESIAN_POINT('',(271.225327339779,118.051631644471,264.903720152625));
#20183=CARTESIAN_POINT('Origin',(267.935464280873,103.783873001336,264.903720152574));
#20184=CARTESIAN_POINT('Origin',(271.225327339779,118.051631644471,264.903720152625));
#20185=CARTESIAN_POINT('',(271.112985016796,117.564415878648,260.32594901942));
#20186=CARTESIAN_POINT('',(271.112985016796,117.564415878648,260.821237247987));
#20187=CARTESIAN_POINT('',(271.112985016796,117.564415878648,264.903720152625));
#20188=CARTESIAN_POINT('Origin',(267.935464280956,103.783873002082,264.90372015265));
#20189=CARTESIAN_POINT('',(270.907762764176,116.674390514045,256.243466114781));
#20190=CARTESIAN_POINT('',(271.225327339779,118.051631644471,256.243466114781));
#20191=CARTESIAN_POINT('Origin',(267.935464280502,103.783873000137,256.243466114489));
#20192=CARTESIAN_POINT('Origin',(271.225327339779,118.051631644471,256.243466114781));
#20193=CARTESIAN_POINT('',(267.66784929765,118.358796062609,254.202224662462));
#20194=CARTESIAN_POINT('',(271.112985016796,117.564415878648,256.243466114781));
#20195=CARTESIAN_POINT('Origin',(267.935464280876,103.783873001347,256.243466114831));
#20196=CARTESIAN_POINT('',(263.917090852433,119.736766489228,251.913339095859));
#20197=CARTESIAN_POINT('Origin',(263.917090852433,119.736766489228,251.913339095859));
#20198=CARTESIAN_POINT('',(256.291289789483,120.044660203559,256.243466114781));
#20199=CARTESIAN_POINT('',(256.608854365086,121.421901333985,256.243466114781));
#20200=CARTESIAN_POINT('',(259.941647761247,120.140305384201,254.202224662462));
#20201=CARTESIAN_POINT('Origin',(253.318991306673,107.154142692754,256.243466114698));
#20202=CARTESIAN_POINT('',(263.804748529449,119.249550723405,251.913339095859));
#20203=CARTESIAN_POINT('Origin',(256.608854365086,121.421901333985,256.243466114781));
#20204=CARTESIAN_POINT('',(256.496512042102,120.934685568162,260.821237247987));
#20205=CARTESIAN_POINT('Origin',(253.318991306164,107.154142691181,264.903720152705));
#20206=CARTESIAN_POINT('',(256.496512042102,120.934685568162,260.32594901942));
#20207=CARTESIAN_POINT('',(256.496512042102,120.934685568162,256.243466114781));
#20208=CARTESIAN_POINT('Origin',(253.31899130647,107.15414269249,256.243466114903));
#20209=CARTESIAN_POINT('Origin',(249.300617877739,123.107036178742,253.073593133703));
#20210=CARTESIAN_POINT('',(257.096169703538,121.309536051521,260.573593133703));
#20211=CARTESIAN_POINT('Origin',(270.876613007385,118.132038275181,264.697107058593));
#20212=CARTESIAN_POINT('Origin',(270.876613007503,118.132038275155,256.450079208744));
#20213=CARTESIAN_POINT('',(270.738012001328,118.163996926934,260.573593133704));
#20214=CARTESIAN_POINT('Origin',(256.957568697313,121.341494703312,256.450079208715));
#20215=CARTESIAN_POINT('Origin',(256.957568697334,121.341494703307,264.69710705868));
#20216=CARTESIAN_POINT('Origin',(246.379666533197,123.780549809431,258.265580431811));
#20217=CARTESIAN_POINT('',(255.562088621698,117.401987874335,269.05363105279));
#20218=CARTESIAN_POINT('Origin',(259.529805709628,120.748387703296,271.255961488578));
#20219=CARTESIAN_POINT('',(265.586365399582,121.687840922005,265.342093607999));
#20220=CARTESIAN_POINT('Origin',(257.096070130909,121.309559011001,253.073593133703));
#20221=CARTESIAN_POINT('',(257.010851567994,121.256276140383,260.573593133703));
#20222=CARTESIAN_POINT('',(259.309178347426,122.693303992497,259.466995116294));
#20223=CARTESIAN_POINT('',(254.858613753559,119.910590352186,259.537334008256));
#20224=CARTESIAN_POINT('Origin',(270.738111573956,118.163973967455,253.073593133703));
#20225=CARTESIAN_POINT('',(270.791394444574,118.078755404539,260.573593133703));
#20226=CARTESIAN_POINT('',(272.137080232772,115.926517590104,259.537334008256));
#20227=CARTESIAN_POINT('',(269.35436659246,120.377082183972,259.466995116294));
#20228=CARTESIAN_POINT('Origin',(252.708784988104,122.321180225069,259.131605835595));
#20229=CARTESIAN_POINT('',(257.787370918632,118.793344694491,253.164983786045));
#20230=CARTESIAN_POINT('Origin',(253.200687254721,122.207757287658,246.141224778829));
#20231=CARTESIAN_POINT('',(264.195008579426,123.913123218939,256.876521230836));
#20232=CARTESIAN_POINT('Origin',(259.161112492359,117.81723196461,263.000245587794));
#20233=CARTESIAN_POINT('Origin',(262.430485695863,112.851978297123,260.573593240362));
#20234=CARTESIAN_POINT('Origin',(260.875334786248,115.075571113603,259.466995116294));
#20235=CARTESIAN_POINT('Origin',(259.643746269855,111.10869307224,259.288708143003));
#20236=CARTESIAN_POINT('Origin',(262.271656097715,112.843043970938,260.573593172734));
#20237=CARTESIAN_POINT('Origin',(264.610689417795,114.214272186285,259.466995116294));
#20238=CARTESIAN_POINT('Origin',(290.197052756605,75.7062702018219,253.073593133703));
#20239=CARTESIAN_POINT('',(261.613491303351,78.6976913251852,230.342590522438));
#20240=CARTESIAN_POINT('',(259.737667058827,79.3576729844988,230.309496805655));
#20241=CARTESIAN_POINT('Ctrl Pts',(261.613491303076,78.6976913253861,230.342590522417));
#20242=CARTESIAN_POINT('Ctrl Pts',(261.012965195301,78.9874393341337,230.31984533521));
#20243=CARTESIAN_POINT('Ctrl Pts',(260.387795558813,79.2077662059219,230.309496805655));
#20244=CARTESIAN_POINT('Ctrl Pts',(259.737667058827,79.3576729844988,230.309496805655));
#20245=CARTESIAN_POINT('',(289.458803205568,72.5045665978414,230.309496805655));
#20246=CARTESIAN_POINT('',(269.82981977108,91.6423159687713,232.848723505596));
#20247=CARTESIAN_POINT('',(292.657884593393,86.3786155484235,232.848723505596));
#20248=CARTESIAN_POINT('Ctrl Pts',(269.82981977108,91.6423159687712,232.848723505596));
#20249=CARTESIAN_POINT('Ctrl Pts',(269.412062867116,91.4518718255699,232.697399160319));
#20250=CARTESIAN_POINT('Ctrl Pts',(269.005494956222,91.2443405944999,232.545799518012));
#20251=CARTESIAN_POINT('Ctrl Pts',(268.609998824741,91.018971085966,232.395516517388));
#20252=CARTESIAN_POINT('Ctrl Pts',(268.222148036074,90.7979581994462,232.248138640147));
#20253=CARTESIAN_POINT('Ctrl Pts',(267.844945108691,90.5597901305427,232.102027006344));
#20254=CARTESIAN_POINT('Ctrl Pts',(267.478273206019,90.3037347924297,231.958726010898));
#20255=CARTESIAN_POINT('Ctrl Pts',(267.137265294114,90.0656012033941,231.82545489611));
#20256=CARTESIAN_POINT('Ctrl Pts',(266.805365789826,89.8119965611551,231.694615072261));
#20257=CARTESIAN_POINT('Ctrl Pts',(266.482475600845,89.5423115743041,231.567483405361));
#20258=CARTESIAN_POINT('Ctrl Pts',(266.463505779451,89.5264675622914,231.560014410957));
#20259=CARTESIAN_POINT('Ctrl Pts',(266.444566559758,89.5105672705819,231.552557898557));
#20260=CARTESIAN_POINT('Ctrl Pts',(266.425658042599,89.4946106679016,231.545114183402));
#20261=CARTESIAN_POINT('Ctrl Pts',(266.224546364397,89.3248956597622,231.465942557493));
#20262=CARTESIAN_POINT('Ctrl Pts',(266.026936720047,89.148522798973,231.388184363742));
#20263=CARTESIAN_POINT('Ctrl Pts',(265.83461601482,88.9669001566157,231.312816009738));
#20264=CARTESIAN_POINT('Ctrl Pts',(265.800972613982,88.9351282090711,231.299631533624));
#20265=CARTESIAN_POINT('Ctrl Pts',(265.767491061666,88.9031957372929,231.286520197391));
#20266=CARTESIAN_POINT('Ctrl Pts',(265.734180908561,88.8711104332793,231.273487229652));
#20267=CARTESIAN_POINT('Ctrl Pts',(265.714141013639,88.8518074262067,231.265646397963));
#20268=CARTESIAN_POINT('Ctrl Pts',(265.69416030416,88.8324465029543,231.257832863114));
#20269=CARTESIAN_POINT('Ctrl Pts',(265.674240936888,88.8130292915668,231.250047785851));
#20270=CARTESIAN_POINT('Ctrl Pts',(265.472975056506,88.6168372092048,231.17138713325));
#20271=CARTESIAN_POINT('Ctrl Pts',(265.277392278449,88.4144325332718,231.095401978004));
#20272=CARTESIAN_POINT('Ctrl Pts',(265.087752747776,88.2057836732551,231.022485409116));
#20273=CARTESIAN_POINT('Ctrl Pts',(265.069859489022,88.1860968071894,231.015605435146));
#20274=CARTESIAN_POINT('Ctrl Pts',(265.052019113926,88.1663543769224,231.008752771387));
#20275=CARTESIAN_POINT('Ctrl Pts',(265.03423182395,88.1465563722257,231.00192774245));
#20276=CARTESIAN_POINT('Ctrl Pts',(265.014562170462,88.1246632174707,230.994380445789));
#20277=CARTESIAN_POINT('Ctrl Pts',(264.994956786706,88.1027013973482,230.986866698014));
#20278=CARTESIAN_POINT('Ctrl Pts',(264.975415760474,88.0806706935066,230.979386876402));
#20279=CARTESIAN_POINT('Ctrl Pts',(264.771466620346,87.850736858316,230.901320189011));
#20280=CARTESIAN_POINT('Ctrl Pts',(264.574526846944,87.6133013235892,230.826946705393));
#20281=CARTESIAN_POINT('Ctrl Pts',(264.384829486875,87.3680005217492,230.756727452304));
#20282=CARTESIAN_POINT('Ctrl Pts',(264.366629531072,87.3444658571115,230.7499904724));
#20283=CARTESIAN_POINT('Ctrl Pts',(264.348495277114,87.3208574571962,230.743291364523));
#20284=CARTESIAN_POINT('Ctrl Pts',(264.330427274506,87.2971753749938,230.73663066703));
#20285=CARTESIAN_POINT('Ctrl Pts',(264.192051910297,87.1158040955474,230.685619137893));
#20286=CARTESIAN_POINT('Ctrl Pts',(264.057307830443,86.9296671023993,230.636776967807));
#20287=CARTESIAN_POINT('Ctrl Pts',(263.927380064349,86.7402318307243,230.590657569167));
#20288=CARTESIAN_POINT('Ctrl Pts',(263.880505355907,86.6718882934231,230.574018836509));
#20289=CARTESIAN_POINT('Ctrl Pts',(263.834257363913,86.6031159271292,230.5577343861));
#20290=CARTESIAN_POINT('Ctrl Pts',(263.788690979733,86.5339850002118,230.541829743817));
#20291=CARTESIAN_POINT('Ctrl Pts',(263.77298301991,86.5101537078662,230.536346985278));
#20292=CARTESIAN_POINT('Ctrl Pts',(263.75735496487,86.4862783657571,230.530909020002));
#20293=CARTESIAN_POINT('Ctrl Pts',(263.741808862961,86.4623615195282,230.525516828383));
#20294=CARTESIAN_POINT('Ctrl Pts',(263.484549544799,86.066581819303,230.436286000791));
#20295=CARTESIAN_POINT('Ctrl Pts',(263.248690603452,85.6584941433215,230.359194420258));
#20296=CARTESIAN_POINT('Ctrl Pts',(263.034697118873,85.2379084504163,230.295174158128));
#20297=CARTESIAN_POINT('Ctrl Pts',(262.951489163286,85.0743704075428,230.270280899633));
#20298=CARTESIAN_POINT('Ctrl Pts',(262.871586616947,84.9089430262691,230.247363811953));
#20299=CARTESIAN_POINT('Ctrl Pts',(262.79501499609,84.7416161629987,230.226477214704));
#20300=CARTESIAN_POINT('Ctrl Pts',(262.785462820506,84.7207424298838,230.223871648281));
#20301=CARTESIAN_POINT('Ctrl Pts',(262.775962440878,84.699838964399,230.221297659614));
#20302=CARTESIAN_POINT('Ctrl Pts',(262.766513896054,84.6789057298734,230.218755353273));
#20303=CARTESIAN_POINT('Ctrl Pts',(262.634811555875,84.3871194256535,230.183318394364));
#20304=CARTESIAN_POINT('Ctrl Pts',(262.513220219422,84.0895305978623,230.154044317955));
#20305=CARTESIAN_POINT('Ctrl Pts',(262.402090716589,83.7859199686843,230.131279947247));
#20306=CARTESIAN_POINT('Ctrl Pts',(262.395546655457,83.7680413094,230.129939426236));
#20307=CARTESIAN_POINT('Ctrl Pts',(262.389038572057,83.7501409057057,230.128621416215));
#20308=CARTESIAN_POINT('Ctrl Pts',(262.382566616886,83.7322188864832,230.127326007806));
#20309=CARTESIAN_POINT('Ctrl Pts',(262.312662251443,83.5386410034226,230.113334145927));
#20310=CARTESIAN_POINT('Ctrl Pts',(262.246832138757,83.3419473504265,230.101977077434));
#20311=CARTESIAN_POINT('Ctrl Pts',(262.185666534111,83.1437789606774,230.093387800197));
#20312=CARTESIAN_POINT('Ctrl Pts',(262.149430174372,83.0263779948678,230.088299251794));
#20313=CARTESIAN_POINT('Ctrl Pts',(262.114830284334,82.908460176112,230.084181676947));
#20314=CARTESIAN_POINT('Ctrl Pts',(262.081982731389,82.7903697894063,230.081058549722));
#20315=CARTESIAN_POINT('Ctrl Pts',(262.078182411074,82.7767072405916,230.080697217362));
#20316=CARTESIAN_POINT('Ctrl Pts',(262.074405587126,82.763042642054,230.080349199255));
#20317=CARTESIAN_POINT('Ctrl Pts',(262.070652408175,82.7493764437098,230.080014525542));
#20318=CARTESIAN_POINT('Ctrl Pts',(261.979457301859,82.417313830294,230.0718825912));
#20319=CARTESIAN_POINT('Ctrl Pts',(261.901916508769,82.0840986416051,230.071504242517));
#20320=CARTESIAN_POINT('Ctrl Pts',(261.837665799815,81.7496382953417,230.078654173433));
#20321=CARTESIAN_POINT('Ctrl Pts',(261.773415090861,81.4151779490784,230.08580410435));
#20322=CARTESIAN_POINT('Ctrl Pts',(261.722454613692,81.0794724258029,230.100482419413));
#20323=CARTESIAN_POINT('Ctrl Pts',(261.684465227673,80.7424242137756,230.12248991823));
#20324=CARTESIAN_POINT('Ctrl Pts',(261.64549555144,80.3966787023512,230.145065305555));
#20325=CARTESIAN_POINT('Ctrl Pts',(261.620197803172,80.0493109343409,230.175394454572));
#20326=CARTESIAN_POINT('Ctrl Pts',(261.608673985579,79.7006034747511,230.213303729148));
#20327=CARTESIAN_POINT('Ctrl Pts',(261.597663923829,79.3674421216154,230.24952292913));
#20328=CARTESIAN_POINT('Ctrl Pts',(261.599227267589,79.0330576316676,230.292661700132));
#20329=CARTESIAN_POINT('Ctrl Pts',(261.613491303076,78.6976913253862,230.342590522417));
#20330=CARTESIAN_POINT('Origin',(290.197052756605,75.7062702018219,253.073593133703));
#20331=CARTESIAN_POINT('',(259.737667058827,79.3576729844988,275.837689461751));
#20332=CARTESIAN_POINT('',(289.458803205568,72.5045665978414,275.837689461751));
#20333=CARTESIAN_POINT('',(261.613491303351,78.6976913251852,275.804595744969));
#20334=CARTESIAN_POINT('Ctrl Pts',(259.737667058827,79.3576729844988,275.837689461751));
#20335=CARTESIAN_POINT('Ctrl Pts',(260.387795558813,79.2077662059219,275.837689461751));
#20336=CARTESIAN_POINT('Ctrl Pts',(261.012965195301,78.9874393341337,275.827340932196));
#20337=CARTESIAN_POINT('Ctrl Pts',(261.613491303076,78.6976913253861,275.804595744989));
#20338=CARTESIAN_POINT('',(269.82981977108,91.6423159687713,273.29846276181));
#20339=CARTESIAN_POINT('Ctrl Pts',(261.613491303076,78.6976913253861,275.804595744989));
#20340=CARTESIAN_POINT('Ctrl Pts',(261.603419886992,78.9344836142266,275.839849018459));
#20341=CARTESIAN_POINT('Ctrl Pts',(261.599669504006,79.1715618901526,275.871823022698));
#20342=CARTESIAN_POINT('Ctrl Pts',(261.602281421227,79.4088047836705,275.900417526435));
#20343=CARTESIAN_POINT('Ctrl Pts',(261.604869397012,79.6438730541296,275.928749926358));
#20344=CARTESIAN_POINT('Ctrl Pts',(261.613703439758,79.8791034159246,275.953764712688));
#20345=CARTESIAN_POINT('Ctrl Pts',(261.628866516772,80.1143982791075,275.975346498954));
#20346=CARTESIAN_POINT('Ctrl Pts',(261.642231690708,80.321793965998,275.994369308575));
#20347=CARTESIAN_POINT('Ctrl Pts',(261.660514524517,80.5292402432758,276.010724810371));
#20348=CARTESIAN_POINT('Ctrl Pts',(261.683801145841,80.7366793730089,276.024320275013));
#20349=CARTESIAN_POINT('Ctrl Pts',(261.685335442275,80.7503470112872,276.025216045705));
#20350=CARTESIAN_POINT('Ctrl Pts',(261.68689089014,80.7640100348414,276.026099586327));
#20351=CARTESIAN_POINT('Ctrl Pts',(261.688467484406,80.7776684911368,276.026970901121));
#20352=CARTESIAN_POINT('Ctrl Pts',(261.721888633146,81.0672048095263,276.045441310387));
#20353=CARTESIAN_POINT('Ctrl Pts',(261.764898719889,81.3553538370425,276.058458227586));
#20354=CARTESIAN_POINT('Ctrl Pts',(261.817479571976,81.6419481819336,276.065959232372));
#20355=CARTESIAN_POINT('Ctrl Pts',(261.82457895601,81.6806437000837,276.066972006253));
#20356=CARTESIAN_POINT('Ctrl Pts',(261.831852749041,81.7193108918648,276.067884263523));
#20357=CARTESIAN_POINT('Ctrl Pts',(261.839300844835,81.7579493597271,276.068695886441));
#20358=CARTESIAN_POINT('Ctrl Pts',(261.842753889475,81.7758627107472,276.069072166533));
#20359=CARTESIAN_POINT('Ctrl Pts',(261.846245375141,81.793772849323,276.069426653246));
#20360=CARTESIAN_POINT('Ctrl Pts',(261.849775083155,81.8116789582788,276.069759361994));
#20361=CARTESIAN_POINT('Ctrl Pts',(261.890544284871,82.018499965865,276.073602249275));
#20362=CARTESIAN_POINT('Ctrl Pts',(261.936461352576,82.2249739958989,276.074541167105));
#20363=CARTESIAN_POINT('Ctrl Pts',(261.987165998336,82.4296701642412,276.072593815571));
#20364=CARTESIAN_POINT('Ctrl Pts',(262.014944591286,82.5418131731036,276.071526957007));
#20365=CARTESIAN_POINT('Ctrl Pts',(262.044159320794,82.6534226072953,276.069594266407));
#20366=CARTESIAN_POINT('Ctrl Pts',(262.074745527312,82.7642652337524,276.066801927027));
#20367=CARTESIAN_POINT('Ctrl Pts',(262.080807575631,82.7862337428924,276.066248497943));
#20368=CARTESIAN_POINT('Ctrl Pts',(262.086923423206,82.8081751913569,276.065661660633));
#20369=CARTESIAN_POINT('Ctrl Pts',(262.093092874244,82.830089346474,276.065041526113));
#20370=CARTESIAN_POINT('Ctrl Pts',(262.239688206997,83.3508022659059,276.050306207561));
#20371=CARTESIAN_POINT('Ctrl Pts',(262.41667027088,83.8566774376446,276.016757809987));
#20372=CARTESIAN_POINT('Ctrl Pts',(262.622710540289,84.3484094919605,275.965660356875));
#20373=CARTESIAN_POINT('Ctrl Pts',(262.669732754181,84.4606318740334,275.95399896963));
#20374=CARTESIAN_POINT('Ctrl Pts',(262.718268563109,84.5721175147771,275.941423440521));
#20375=CARTESIAN_POINT('Ctrl Pts',(262.768302408475,84.6828744721218,275.927948585287));
#20376=CARTESIAN_POINT('Ctrl Pts',(262.780537482962,84.7099585311849,275.924653498605));
#20377=CARTESIAN_POINT('Ctrl Pts',(262.79286252355,84.7369988532753,275.921304525794));
#20378=CARTESIAN_POINT('Ctrl Pts',(262.805277497977,84.7639954743981,275.917901836472));
#20379=CARTESIAN_POINT('Ctrl Pts',(262.911345432536,84.994642412861,275.888830795653));
#20380=CARTESIAN_POINT('Ctrl Pts',(263.024017624507,85.2221756769784,275.855827045657));
#20381=CARTESIAN_POINT('Ctrl Pts',(263.143170912963,85.446437155884,275.819023904925));
#20382=CARTESIAN_POINT('Ctrl Pts',(263.169270686232,85.4955602126477,275.810962410012));
#20383=CARTESIAN_POINT('Ctrl Pts',(263.195681264233,85.5445263664599,275.802718709764));
#20384=CARTESIAN_POINT('Ctrl Pts',(263.222401085225,85.593334085818,275.794294354551));
#20385=CARTESIAN_POINT('Ctrl Pts',(263.237950817452,85.6217379799495,275.78939175929));
#20386=CARTESIAN_POINT('Ctrl Pts',(263.253611058094,85.6500969358685,275.784425951054));
#20387=CARTESIAN_POINT('Ctrl Pts',(263.269379805331,85.6784078046249,275.779397861218));
#20388=CARTESIAN_POINT('Ctrl Pts',(263.369197762317,85.8576188121514,275.747569482756));
#20389=CARTESIAN_POINT('Ctrl Pts',(263.473528417736,86.0351791520541,275.71319386757));
#20390=CARTESIAN_POINT('Ctrl Pts',(263.581823584891,86.2101512509082,275.67651972138));
#20391=CARTESIAN_POINT('Ctrl Pts',(263.636102278675,86.2978491346089,275.658138247828));
#20392=CARTESIAN_POINT('Ctrl Pts',(263.691376235654,86.384897129559,275.639179737817));
#20393=CARTESIAN_POINT('Ctrl Pts',(263.747572835325,86.4711798102641,275.619677600556));
#20394=CARTESIAN_POINT('Ctrl Pts',(263.766352924537,86.5000142317514,275.613160268907));
#20395=CARTESIAN_POINT('Ctrl Pts',(263.785222875216,86.5287501659856,275.60658677669));
#20396=CARTESIAN_POINT('Ctrl Pts',(263.804181798426,86.5573870000339,275.599957983946));
#20397=CARTESIAN_POINT('Ctrl Pts',(263.99926400509,86.8520522991073,275.531749494383));
#20398=CARTESIAN_POINT('Ctrl Pts',(264.203747945169,87.1363444639111,275.457666020119));
#20399=CARTESIAN_POINT('Ctrl Pts',(264.417436929835,87.4107743914387,275.378347943292));
#20400=CARTESIAN_POINT('Ctrl Pts',(264.635378479409,87.6906656724454,275.297451379531));
#20401=CARTESIAN_POINT('Ctrl Pts',(264.862895108527,87.9602981495343,275.211109589539));
#20402=CARTESIAN_POINT('Ctrl Pts',(265.099806030715,88.2201770788809,275.119971097024));
#20403=CARTESIAN_POINT('Ctrl Pts',(265.34425799555,88.488328138829,275.025931601665));
#20404=CARTESIAN_POINT('Ctrl Pts',(265.598711781157,88.7460947841456,274.926785005734));
#20405=CARTESIAN_POINT('Ctrl Pts',(265.862998468363,88.993994667417,274.823214078989));
#20406=CARTESIAN_POINT('Ctrl Pts',(266.044076214604,89.1638448881395,274.752251783501));
#20407=CARTESIAN_POINT('Ctrl Pts',(266.22977053553,89.3290624729336,274.679211910719));
#20408=CARTESIAN_POINT('Ctrl Pts',(266.420034893768,89.4898045719229,274.604307092073));
#20409=CARTESIAN_POINT('Ctrl Pts',(266.441020935556,89.5075343266592,274.596045136609));
#20410=CARTESIAN_POINT('Ctrl Pts',(266.462047068505,89.5251961709156,274.587766503733));
#20411=CARTESIAN_POINT('Ctrl Pts',(266.483113285084,89.5427902642426,274.579471564047));
#20412=CARTESIAN_POINT('Ctrl Pts',(266.739576892666,89.7569836686354,274.47848759531));
#20413=CARTESIAN_POINT('Ctrl Pts',(267.001631199948,89.9608895027467,274.375211039575));
#20414=CARTESIAN_POINT('Ctrl Pts',(267.269275334688,90.1548901204229,274.270292993316));
#20415=CARTESIAN_POINT('Ctrl Pts',(267.540201437032,90.3512696571924,274.164088396806));
#20416=CARTESIAN_POINT('Ctrl Pts',(267.816855288512,90.537499489122,274.056201405317));
#20417=CARTESIAN_POINT('Ctrl Pts',(268.099260614184,90.7139333766602,273.94728207569));
#20418=CARTESIAN_POINT('Ctrl Pts',(268.389137035801,90.8950348620868,273.835481260879));
#20419=CARTESIAN_POINT('Ctrl Pts',(268.685073201994,91.0658152717133,273.722592360192));
#20420=CARTESIAN_POINT('Ctrl Pts',(268.98712122822,91.2266125215922,273.609298017563));
#20421=CARTESIAN_POINT('Ctrl Pts',(269.262905643181,91.3734281655784,273.505854818842));
#20422=CARTESIAN_POINT('Ctrl Pts',(269.543785584644,91.5119206718048,273.402073104508));
#20423=CARTESIAN_POINT('Ctrl Pts',(269.82981977108,91.6423159687712,273.29846276181));
#20424=CARTESIAN_POINT('',(292.657884593393,86.3786155484235,273.29846276181));
#20425=CARTESIAN_POINT('Origin',(255.074370622327,80.7261481941816,260.573593133704));
#20426=CARTESIAN_POINT('Origin',(139.64640668573,110.42027268846,253.073593133703));
#20427=CARTESIAN_POINT('Origin',(289.522998818702,72.7829756068832,273.85820282453));
#20428=CARTESIAN_POINT('Origin',(259.80186267196,79.6360819935406,273.85820282453));
#20429=CARTESIAN_POINT('Ctrl Pts',(259.352493380025,77.6872189302482,273.85820282453));
#20430=CARTESIAN_POINT('Ctrl Pts',(259.352493380025,77.6872189302482,275.590253632099));
#20431=CARTESIAN_POINT('Ctrl Pts',(259.737667058827,79.3576729844988,275.837689461751));
#20432=CARTESIAN_POINT('Ctrl Pts',(259.950395610532,77.5493544968614,273.858202824316));
#20433=CARTESIAN_POINT('Ctrl Pts',(259.969638708473,77.5449174176954,275.590253631842));
#20434=CARTESIAN_POINT('Ctrl Pts',(260.489866638764,79.1842306313116,275.837689461527));
#20435=CARTESIAN_POINT('Ctrl Pts',(260.520304163086,77.34418247573,273.845727756372));
#20436=CARTESIAN_POINT('Ctrl Pts',(260.55632630418,77.3317737998276,275.572104967451));
#20437=CARTESIAN_POINT('Ctrl Pts',(261.204913401109,78.9177192700401,275.824026291386));
#20438=CARTESIAN_POINT('Ctrl Pts',(261.334314889648,76.9392458488615,273.803773140294));
#20439=CARTESIAN_POINT('Ctrl Pts',(261.39984718193,76.9039004839026,275.514566262518));
#20440=CARTESIAN_POINT('Ctrl Pts',(262.223292632644,78.3835679167525,275.778075998304));
#20441=CARTESIAN_POINT('Ctrl Pts',(261.600168265855,76.7869681618089,273.78564891822));
#20442=CARTESIAN_POINT('Ctrl Pts',(261.675379825811,76.7425527899067,275.490123794013));
#20443=CARTESIAN_POINT('Ctrl Pts',(262.555366780798,78.1816425648451,275.758225659285));
#20444=CARTESIAN_POINT('Ctrl Pts',(262.110942369245,76.4526422432437,273.739442671591));
#20445=CARTESIAN_POINT('Ctrl Pts',(262.205789159906,76.3857612367168,275.429609986423));
#20446=CARTESIAN_POINT('Ctrl Pts',(263.192272886497,77.7364025768395,275.707618818374));
#20447=CARTESIAN_POINT('Ctrl Pts',(262.353991061074,76.2720769658325,273.711582345508));
#20448=CARTESIAN_POINT('Ctrl Pts',(262.458640311379,76.1920833314006,275.393879863165));
#20449=CARTESIAN_POINT('Ctrl Pts',(263.494777280233,77.4950731950082,275.67710512717));
#20450=CARTESIAN_POINT('Ctrl Pts',(262.816166800432,75.8852869421232,273.643922776295));
#20451=CARTESIAN_POINT('Ctrl Pts',(262.93982714268,75.7742357891089,275.309622118513));
#20452=CARTESIAN_POINT('Ctrl Pts',(264.068873292152,76.9765864414364,275.603001790289));
#20453=CARTESIAN_POINT('Ctrl Pts',(263.035290733386,75.6790579795937,273.604129294606));
#20454=CARTESIAN_POINT('Ctrl Pts',(263.168240525528,75.5501498442423,275.261138675086));
#20455=CARTESIAN_POINT('Ctrl Pts',(264.340460862288,76.6994232039232,275.559418452284));
#20456=CARTESIAN_POINT('Ctrl Pts',(263.449407025878,75.2411080436662,273.509217640416));
#20457=CARTESIAN_POINT('Ctrl Pts',(263.599273270717,75.0709585050466,275.148629692437));
#20458=CARTESIAN_POINT('Ctrl Pts',(264.852462244811,76.1094929549171,275.455467593939));
#20459=CARTESIAN_POINT('Ctrl Pts',(263.645621061591,75.0075891196608,273.453599168673));
#20460=CARTESIAN_POINT('Ctrl Pts',(263.803351197742,74.8137915708697,275.084050570573));
#20461=CARTESIAN_POINT('Ctrl Pts',(265.094373229636,75.7942915062644,275.394552123933));
#20462=CARTESIAN_POINT('Ctrl Pts',(264.18452429865,74.2844949805711,273.261503260181));
#20463=CARTESIAN_POINT('Ctrl Pts',(264.360159533119,74.0132571206072,274.86652779898));
#20464=CARTESIAN_POINT('Ctrl Pts',(265.756639414063,74.8164649195017,275.184161368368));
#20465=CARTESIAN_POINT('Ctrl Pts',(264.479839828946,73.7723884511662,273.100414005911));
#20466=CARTESIAN_POINT('Ctrl Pts',(264.662785788954,73.4369654880319,274.689319013975));
#20467=CARTESIAN_POINT('Ctrl Pts',(266.116520847396,74.1216801997296,275.007727891442));
#20468=CARTESIAN_POINT('Ctrl Pts',(264.714335805196,73.2350168556771,272.892880023885));
#20469=CARTESIAN_POINT('Ctrl Pts',(264.891797790303,72.8283445041923,274.469890825203));
#20470=CARTESIAN_POINT('Ctrl Pts',(266.39885077907,73.3906559987533,274.780431156283));
#20471=CARTESIAN_POINT('Ctrl Pts',(261.613491303169,78.6976913251228,275.804595744953));
#20472=CARTESIAN_POINT('Ctrl Pts',(261.640463121467,78.6217294719184,275.79410972222));
#20473=CARTESIAN_POINT('Ctrl Pts',(261.668927419666,78.5471358444608,275.781382564128));
#20474=CARTESIAN_POINT('Ctrl Pts',(261.698675179246,78.4737068307562,275.76674155216));
#20475=CARTESIAN_POINT('Ctrl Pts',(261.729027718461,78.3987849862377,275.751802884637));
#20476=CARTESIAN_POINT('Ctrl Pts',(261.76071647419,78.3250757793365,275.734871638552));
#20477=CARTESIAN_POINT('Ctrl Pts',(261.793541102325,78.2523960866447,275.716256908152));
#20478=CARTESIAN_POINT('Ctrl Pts',(261.827408822181,78.1774067992964,275.697050644129));
#20479=CARTESIAN_POINT('Ctrl Pts',(261.862485754497,78.1035136413755,275.676052146321));
#20480=CARTESIAN_POINT('Ctrl Pts',(261.89857443723,78.0305479237867,275.653561505271));
#20481=CARTESIAN_POINT('Ctrl Pts',(261.916261738067,77.9947869455509,275.642538694125));
#20482=CARTESIAN_POINT('Ctrl Pts',(261.934192403458,77.9592492137772,275.63115687955));
#20483=CARTESIAN_POINT('Ctrl Pts',(261.952345067313,77.9239174154688,275.619448165681));
#20484=CARTESIAN_POINT('Ctrl Pts',(261.985756831217,77.8588857643113,275.597897125759));
#20485=CARTESIAN_POINT('Ctrl Pts',(262.01988412855,77.794622083521,275.575265396718));
#20486=CARTESIAN_POINT('Ctrl Pts',(262.054660477631,77.7309198561505,275.55169804487));
#20487=CARTESIAN_POINT('Ctrl Pts',(262.090751989985,77.6648085538752,275.527239428803));
#20488=CARTESIAN_POINT('Ctrl Pts',(262.127542591829,77.5993022921848,275.501772939713));
#20489=CARTESIAN_POINT('Ctrl Pts',(262.164991025203,77.5341799597694,275.475416808112));
#20490=CARTESIAN_POINT('Ctrl Pts',(262.173788840419,77.5188806749813,275.469224923572));
#20491=CARTESIAN_POINT('Ctrl Pts',(262.182623101299,77.5036026092372,275.462983758236));
#20492=CARTESIAN_POINT('Ctrl Pts',(262.191493522389,77.4883429401822,275.456694524797));
#20493=CARTESIAN_POINT('Ctrl Pts',(262.231953816496,77.418739626913,275.428007697861));
#20494=CARTESIAN_POINT('Ctrl Pts',(262.272838079584,77.350048000437,275.398535810711));
#20495=CARTESIAN_POINT('Ctrl Pts',(262.314099531327,77.2819808754804,275.368314912438));
#20496=CARTESIAN_POINT('Ctrl Pts',(262.328401654566,77.258387318577,275.357839686938));
#20497=CARTESIAN_POINT('Ctrl Pts',(262.342749438049,77.2348688922053,275.347274161733));
#20498=CARTESIAN_POINT('Ctrl Pts',(262.357141963554,77.2114139037108,275.336618888011));
#20499=CARTESIAN_POINT('Ctrl Pts',(262.410079203,77.1251439616009,275.297427658077));
#20500=CARTESIAN_POINT('Ctrl Pts',(262.463569962561,77.0398179251102,275.257065801432));
#20501=CARTESIAN_POINT('Ctrl Pts',(262.517379093069,76.9552242466752,275.215708031544));
#20502=CARTESIAN_POINT('Ctrl Pts',(262.572627824017,76.8683673631756,275.173243782827));
#20503=CARTESIAN_POINT('Ctrl Pts',(262.628212404354,76.7822827727532,275.129729548656));
#20504=CARTESIAN_POINT('Ctrl Pts',(262.683920945102,76.6967676750229,275.085326562061));
#20505=CARTESIAN_POINT('Ctrl Pts',(262.742307773582,76.6071412860253,275.038788822471));
#20506=CARTESIAN_POINT('Ctrl Pts',(262.800830872367,76.518140639542,274.991274835981));
#20507=CARTESIAN_POINT('Ctrl Pts',(262.85929021809,76.4295576324981,274.942940292671));
#20508=CARTESIAN_POINT('Ctrl Pts',(262.908026182039,76.3557083927509,274.90264510067));
#20509=CARTESIAN_POINT('Ctrl Pts',(262.956718746885,76.2821499717718,274.861779015391));
#20510=CARTESIAN_POINT('Ctrl Pts',(263.005272555425,76.2087727973901,274.820417589951));
#20511=CARTESIAN_POINT('Ctrl Pts',(263.060542637539,76.1252456225852,274.773334787403));
#20512=CARTESIAN_POINT('Ctrl Pts',(263.115708369896,76.0418382064472,274.725490781205));
#20513=CARTESIAN_POINT('Ctrl Pts',(263.170530251593,75.958601926688,274.677015542267));
#20514=CARTESIAN_POINT('Ctrl Pts',(263.18715735304,75.9333569328139,274.662313334125));
#20515=CARTESIAN_POINT('Ctrl Pts',(263.203753124808,75.9081275516313,274.647552890128));
#20516=CARTESIAN_POINT('Ctrl Pts',(263.220311635213,75.8829148882721,274.632737403038));
#20517=CARTESIAN_POINT('Ctrl Pts',(263.280731719076,75.7909168040654,274.578677409079));
#20518=CARTESIAN_POINT('Ctrl Pts',(263.340785418365,75.6989423502989,274.523770259114));
#20519=CARTESIAN_POINT('Ctrl Pts',(263.400202842949,75.6070406003285,274.468146294033));
#20520=CARTESIAN_POINT('Ctrl Pts',(263.417872769097,75.5797102818875,274.451604490649));
#20521=CARTESIAN_POINT('Ctrl Pts',(263.4354867097,75.5523862658522,274.434999122649));
#20522=CARTESIAN_POINT('Ctrl Pts',(263.453038257251,75.5250695291328,274.418333198669));
#20523=CARTESIAN_POINT('Ctrl Pts',(263.531183974767,75.4034457244507,274.344130591536));
#20524=CARTESIAN_POINT('Ctrl Pts',(263.60801194364,75.2820831684112,274.268811207293));
#20525=CARTESIAN_POINT('Ctrl Pts',(263.683293494855,75.1607510839154,274.192319481584));
#20526=CARTESIAN_POINT('Ctrl Pts',(263.756243034221,75.0431775279582,274.118197255543));
#20527=CARTESIAN_POINT('Ctrl Pts',(263.827741740394,74.9256328135397,274.042974155082));
#20528=CARTESIAN_POINT('Ctrl Pts',(263.897622681191,74.8078999833618,273.966578931842));
#20529=CARTESIAN_POINT('Ctrl Pts',(263.941871575824,74.7333510786387,273.918205167192));
#20530=CARTESIAN_POINT('Ctrl Pts',(263.985462003184,74.6587045073954,273.869359764373));
#20531=CARTESIAN_POINT('Ctrl Pts',(264.028363007675,74.583948413358,273.820012956539));
#20532=CARTESIAN_POINT('Ctrl Pts',(264.106301190796,74.4481391423252,273.730364693264));
#20533=CARTESIAN_POINT('Ctrl Pts',(264.181908511619,74.3120674435541,273.639133544911));
#20534=CARTESIAN_POINT('Ctrl Pts',(264.25497364732,74.1757277968292,273.54618930162));
#20535=CARTESIAN_POINT('Ctrl Pts',(264.298661947877,74.0942053660987,273.490614560029));
#20536=CARTESIAN_POINT('Ctrl Pts',(264.341442030647,74.0125863394151,273.434426941907));
#20537=CARTESIAN_POINT('Ctrl Pts',(264.383272984049,73.9308629539767,273.377594728271));
#20538=CARTESIAN_POINT('Ctrl Pts',(264.432025871625,73.8356164750296,273.311358262288));
#20539=CARTESIAN_POINT('Ctrl Pts',(264.479623489581,73.7399603004325,273.244059730206));
#20540=CARTESIAN_POINT('Ctrl Pts',(264.525812267634,73.644243708693,273.175895849824));
#20541=CARTESIAN_POINT('Ctrl Pts',(264.571084485189,73.5504264970762,273.109084599295));
#20542=CARTESIAN_POINT('Ctrl Pts',(264.615002988964,73.4565515061618,273.041442047184));
#20543=CARTESIAN_POINT('Ctrl Pts',(264.657365195295,73.3629565418885,272.973187172579));
#20544=CARTESIAN_POINT('Ctrl Pts',(264.670885765522,73.3330842241583,272.951402546487));
#20545=CARTESIAN_POINT('Ctrl Pts',(264.684248094534,73.3032404851218,272.929555803375));
#20546=CARTESIAN_POINT('Ctrl Pts',(264.697446445794,73.2734364402348,272.907654791342));
#20547=CARTESIAN_POINT('Ctrl Pts',(263.544486310321,78.4442745295379,277.78120466771));
#20548=CARTESIAN_POINT('Ctrl Pts',(263.538250261041,78.7291375341272,275.876052151847));
#20549=CARTESIAN_POINT('Ctrl Pts',(261.613491303076,78.6976913253861,275.804595744989));
#20550=CARTESIAN_POINT('Ctrl Pts',(263.557302515182,77.8588297294296,277.680650907661));
#20551=CARTESIAN_POINT('Ctrl Pts',(263.533654545806,78.3947691062696,275.950105354397));
#20552=CARTESIAN_POINT('Ctrl Pts',(261.754727069594,78.2999231642985,275.749686526725));
#20553=CARTESIAN_POINT('Ctrl Pts',(263.606591880381,77.3148820941794,277.451481936637));
#20554=CARTESIAN_POINT('Ctrl Pts',(263.538547887186,77.9742246260938,275.962292428753));
#20555=CARTESIAN_POINT('Ctrl Pts',(261.949245797882,77.9050773398094,275.628452153648));
#20556=CARTESIAN_POINT('Ctrl Pts',(263.755975405511,76.2858158960412,276.814036792249));
#20557=CARTESIAN_POINT('Ctrl Pts',(263.624571850212,77.0153725191991,275.757092055883));
#20558=CARTESIAN_POINT('Ctrl Pts',(262.433710331132,77.0716088320336,275.284928037322));
#20559=CARTESIAN_POINT('Ctrl Pts',(263.852404590492,75.824998225666,276.4197615986));
#20560=CARTESIAN_POINT('Ctrl Pts',(263.698661733633,76.5115820479287,275.559759849144));
#20561=CARTESIAN_POINT('Ctrl Pts',(262.711999049714,76.6519825800893,275.070246533072));
#20562=CARTESIAN_POINT('Ctrl Pts',(264.014706007828,75.1891126872895,275.756206976135));
#20563=CARTESIAN_POINT('Ctrl Pts',(263.858168373587,75.7622723596492,275.132856736245));
#20564=CARTESIAN_POINT('Ctrl Pts',(263.151909041545,75.9871679741537,274.69550296854));
#20565=CARTESIAN_POINT('Ctrl Pts',(264.072112191271,74.9857513363534,275.521600607894));
#20566=CARTESIAN_POINT('Ctrl Pts',(263.917768744914,75.5167006386421,274.972965619438));
#20567=CARTESIAN_POINT('Ctrl Pts',(263.302835955358,75.7588393827117,274.560956346748));
#20568=CARTESIAN_POINT('Ctrl Pts',(264.190557682099,74.5984025565768,275.035373464112));
#20569=CARTESIAN_POINT('Ctrl Pts',(264.048271575533,75.0381564136266,274.623431382325));
#20570=CARTESIAN_POINT('Ctrl Pts',(263.603229270736,75.2913050055039,274.275702018227));
#20571=CARTESIAN_POINT('Ctrl Pts',(264.251478238831,74.4146529473688,274.784242803635));
#20572=CARTESIAN_POINT('Ctrl Pts',(264.119123197892,74.8037832321255,274.43390177169));
#20573=CARTESIAN_POINT('Ctrl Pts',(263.752412397567,75.0525305312594,274.125297564039));
#20574=CARTESIAN_POINT('Ctrl Pts',(264.437749904692,73.8878858378157,274.010861079826));
#20575=CARTESIAN_POINT('Ctrl Pts',(264.343108315133,74.1265992212334,273.83709802127));
#20576=CARTESIAN_POINT('Ctrl Pts',(264.188012233111,74.3186632559562,273.649114033831));
#20577=CARTESIAN_POINT('Ctrl Pts',(264.566427694471,73.5692983043154,273.468513234698));
#20578=CARTESIAN_POINT('Ctrl Pts',(264.514363032585,73.6868688639712,273.383107148469));
#20579=CARTESIAN_POINT('Ctrl Pts',(264.462022086354,73.8050633190648,273.298312058746));
#20580=CARTESIAN_POINT('Ctrl Pts',(264.697446473732,73.2734363771458,272.907654744982));
#20581=CARTESIAN_POINT('Ctrl Pts',(264.697446473732,73.2734363771458,272.907654744982));
#20582=CARTESIAN_POINT('Ctrl Pts',(264.697446473732,73.2734363771458,272.907654744982));
#20583=CARTESIAN_POINT('Origin',(261.544965371427,78.4005022217613,277.78120466771));
#20584=CARTESIAN_POINT('Ctrl Pts',(261.613491303076,78.6976913253861,275.804595744989));
#20585=CARTESIAN_POINT('Ctrl Pts',(263.538250261041,78.7291375341272,275.876052151847));
#20586=CARTESIAN_POINT('Ctrl Pts',(263.544486310321,78.4442745295379,277.78120466771));
#20587=CARTESIAN_POINT('Ctrl Pts',(261.584924963991,79.3693236611784,275.90458733896));
#20588=CARTESIAN_POINT('Ctrl Pts',(263.538751417713,79.3208320667281,275.951422448941));
#20589=CARTESIAN_POINT('Ctrl Pts',(263.530633522654,79.0770704776892,277.889891267409));
#20590=CARTESIAN_POINT('Ctrl Pts',(261.606888594957,80.0515359965378,275.97941629239));
#20591=CARTESIAN_POINT('Ctrl Pts',(263.577708183242,79.9084748007003,276.005543753781));
#20592=CARTESIAN_POINT('Ctrl Pts',(263.561159360681,79.7206789971068,277.971227001875));
#20593=CARTESIAN_POINT('Ctrl Pts',(261.722256160334,81.0792512150198,276.046772257573));
#20594=CARTESIAN_POINT('Ctrl Pts',(263.694408709898,80.7915012776091,276.054308283014));
#20595=CARTESIAN_POINT('Ctrl Pts',(263.679123147862,80.6916047864155,278.044440007458));
#20596=CARTESIAN_POINT('Ctrl Pts',(261.774083994414,81.4196746921591,276.061590187108));
#20597=CARTESIAN_POINT('Ctrl Pts',(263.742807893208,81.0834999396488,276.064954230829));
#20598=CARTESIAN_POINT('Ctrl Pts',(263.730106477294,81.0134428912567,278.060546452654));
#20599=CARTESIAN_POINT('Ctrl Pts',(261.904506161914,82.0962262854197,276.075801577687));
#20600=CARTESIAN_POINT('Ctrl Pts',(263.858611890859,81.6646469545893,276.07518727214));
#20601=CARTESIAN_POINT('Ctrl Pts',(263.855417008547,81.6535129221044,278.075993616262));
#20602=CARTESIAN_POINT('Ctrl Pts',(261.983448859087,82.4334104511011,276.075136798143));
#20603=CARTESIAN_POINT('Ctrl Pts',(263.926196279394,81.9540846684519,276.074711158139));
#20604=CARTESIAN_POINT('Ctrl Pts',(263.930066466954,81.9727463532846,278.075271029728));
#20605=CARTESIAN_POINT('Ctrl Pts',(262.257324061002,83.4259788289607,276.050132170168));
#20606=CARTESIAN_POINT('Ctrl Pts',(264.155346427456,82.8090535366488,276.056711404079));
#20607=CARTESIAN_POINT('Ctrl Pts',(264.186108538369,82.9131611918406,278.048092086594));
#20608=CARTESIAN_POINT('Ctrl Pts',(262.489246294873,84.0651482976787,276.003102117324));
#20609=CARTESIAN_POINT('Ctrl Pts',(264.342254943422,83.3613811113261,276.023184668261));
#20610=CARTESIAN_POINT('Ctrl Pts',(264.399590570473,83.519667383898,277.996972463593));
#20611=CARTESIAN_POINT('Ctrl Pts',(262.907828258109,84.991738509739,275.890371770625));
#20612=CARTESIAN_POINT('Ctrl Pts',(264.679770033545,84.1792123901588,275.94003272305));
#20613=CARTESIAN_POINT('Ctrl Pts',(264.781126806292,84.4002721698412,277.874439478249));
#20614=CARTESIAN_POINT('Ctrl Pts',(263.05918892757,85.2952200573854,275.845750061578));
#20615=CARTESIAN_POINT('Ctrl Pts',(264.801019872423,84.4481788348286,275.907041959933));
#20616=CARTESIAN_POINT('Ctrl Pts',(264.918568019719,84.6889288671942,277.825937620468));
#20617=CARTESIAN_POINT('Ctrl Pts',(263.385603217161,85.8914532581418,275.742838213459));
#20618=CARTESIAN_POINT('Ctrl Pts',(265.063276334391,84.9817577086832,275.829892444549));
#20619=CARTESIAN_POINT('Ctrl Pts',(265.21399891031,85.2565181212866,277.714076916101));
#20620=CARTESIAN_POINT('Ctrl Pts',(263.56129340771,86.1851653448694,275.68432430288));
#20621=CARTESIAN_POINT('Ctrl Pts',(265.204448884394,85.2468357118572,275.785699044745));
#20622=CARTESIAN_POINT('Ctrl Pts',(265.37256137918,85.536366807698,277.650474839131));
#20623=CARTESIAN_POINT('Ctrl Pts',(264.492544874104,87.615324849741,275.361080258794));
#20624=CARTESIAN_POINT('Ctrl Pts',(265.947933666804,86.5352397777713,275.540942276622));
#20625=CARTESIAN_POINT('Ctrl Pts',(266.21092639465,86.9002782684925,277.299122618297));
#20626=CARTESIAN_POINT('Ctrl Pts',(265.38578794737,88.6160477178875,275.011475602805));
#20627=CARTESIAN_POINT('Ctrl Pts',(266.671873010809,87.488473601431,275.267004329307));
#20628=CARTESIAN_POINT('Ctrl Pts',(267.008921214875,87.858651988119,276.919117556122));
#20629=CARTESIAN_POINT('Ctrl Pts',(267.454181512283,90.3636586447312,274.197111457415));
#20630=CARTESIAN_POINT('Ctrl Pts',(268.432540806735,89.2203249048919,274.579653206379));
#20631=CARTESIAN_POINT('Ctrl Pts',(268.84731196028,89.5407379995528,276.033939138256));
#20632=CARTESIAN_POINT('Ctrl Pts',(268.591652650856,91.0778688607264,273.746964814108));
#20633=CARTESIAN_POINT('Ctrl Pts',(269.421598796566,89.9678036643426,274.184725204187));
#20634=CARTESIAN_POINT('Ctrl Pts',(269.854099200818,90.2329609402673,275.544696281663));
#20635=CARTESIAN_POINT('Ctrl Pts',(269.82981977108,91.6423159687712,273.29846276181));
#20636=CARTESIAN_POINT('Ctrl Pts',(270.548229297884,90.584148594095,273.76942958616));
#20637=CARTESIAN_POINT('Ctrl Pts',(270.946701599761,90.7857513677001,275.057147077298));
#20638=CARTESIAN_POINT('Origin',(270.043805148192,92.5703459989105,275.057147077298));
#20639=CARTESIAN_POINT('Origin',(292.443899216281,85.4505855182842,271.539778446323));
#20640=CARTESIAN_POINT('Ctrl Pts',(273.255484225105,91.9275333837837,271.539778446323));
#20641=CARTESIAN_POINT('Ctrl Pts',(273.255484225105,91.9275333837837,271.563577454831));
#20642=CARTESIAN_POINT('Ctrl Pts',(273.253623088777,91.9275219541507,271.587173031064));
#20643=CARTESIAN_POINT('Ctrl Pts',(273.250054608046,91.9274970401005,271.610445617562));
#20644=CARTESIAN_POINT('Ctrl Pts',(273.246348308204,91.927471163839,271.634617019954));
#20645=CARTESIAN_POINT('Ctrl Pts',(273.240800633766,91.9274306765218,271.658439833613));
#20646=CARTESIAN_POINT('Ctrl Pts',(273.233641995375,91.9273743226171,271.681785099849));
#20647=CARTESIAN_POINT('Ctrl Pts',(273.225930813326,91.9273136190035,271.706932284006));
#20648=CARTESIAN_POINT('Ctrl Pts',(273.216350735339,91.9272344125153,271.731525078663));
#20649=CARTESIAN_POINT('Ctrl Pts',(273.205250501302,91.9271376093613,271.755411612847));
#20650=CARTESIAN_POINT('Ctrl Pts',(273.200790481524,91.9270987143272,271.765009105523));
#20651=CARTESIAN_POINT('Ctrl Pts',(273.196085663662,91.9270570129215,271.774492703576));
#20652=CARTESIAN_POINT('Ctrl Pts',(273.191160878823,91.9270127136269,271.7838530879));
#20653=CARTESIAN_POINT('Ctrl Pts',(273.179023642191,91.9269035370763,271.806921953493));
#20654=CARTESIAN_POINT('Ctrl Pts',(273.165569387512,91.926771118345,271.829276213771));
#20655=CARTESIAN_POINT('Ctrl Pts',(273.15105536297,91.9266146820572,271.850962154885));
#20656=CARTESIAN_POINT('Ctrl Pts',(273.144635935929,91.9265454916454,271.860553658356));
#20657=CARTESIAN_POINT('Ctrl Pts',(273.138008484825,91.9264716106079,271.870014436442));
#20658=CARTESIAN_POINT('Ctrl Pts',(273.131192071431,91.9263930063714,271.879348530148));
#20659=CARTESIAN_POINT('Ctrl Pts',(273.114779367358,91.9262037414313,271.901823358029));
#20660=CARTESIAN_POINT('Ctrl Pts',(273.097470710609,91.9259860378421,271.923396697541));
#20661=CARTESIAN_POINT('Ctrl Pts',(273.079474058163,91.9257382169349,271.944193936758));
#20662=CARTESIAN_POINT('Ctrl Pts',(273.066824949306,91.9255640337837,271.958811463188));
#20663=CARTESIAN_POINT('Ctrl Pts',(273.053834764524,91.9253749968506,271.973045197809));
#20664=CARTESIAN_POINT('Ctrl Pts',(273.040561221661,91.9251707917529,271.986933965451));
#20665=CARTESIAN_POINT('Ctrl Pts',(273.018634156517,91.9248334576647,272.009877343566));
#20666=CARTESIAN_POINT('Ctrl Pts',(272.995835208372,91.9244531801533,272.031985181632));
#20667=CARTESIAN_POINT('Ctrl Pts',(272.972361860486,91.9240268228059,272.053385779335));
#20668=CARTESIAN_POINT('Ctrl Pts',(272.947379075074,91.9235730488419,272.076162527787));
#20669=CARTESIAN_POINT('Ctrl Pts',(272.921632200933,91.9230671060948,272.098138107484));
#20670=CARTESIAN_POINT('Ctrl Pts',(272.895300190888,91.922505597192,272.119448758397));
#20671=CARTESIAN_POINT('Ctrl Pts',(272.869453101371,91.9219544288288,272.140366960269));
#20672=CARTESIAN_POINT('Ctrl Pts',(272.843041414019,91.9213497496453,272.160644248366));
#20673=CARTESIAN_POINT('Ctrl Pts',(272.816187852709,91.9206882763742,272.180394894944));
#20674=CARTESIAN_POINT('Ctrl Pts',(272.784505150081,91.9199078487541,272.203697348387));
#20675=CARTESIAN_POINT('Ctrl Pts',(272.752284224801,91.9190489558682,272.226182712055));
#20676=CARTESIAN_POINT('Ctrl Pts',(272.719622978659,91.9181105303922,272.247986020648));
#20677=CARTESIAN_POINT('Ctrl Pts',(272.695125012398,91.9174066529115,272.264339858342));
#20678=CARTESIAN_POINT('Ctrl Pts',(272.670377979989,91.9166579929307,272.28030961091));
#20679=CARTESIAN_POINT('Ctrl Pts',(272.645405122023,91.9158632887775,272.295946522169));
#20680=CARTESIAN_POINT('Ctrl Pts',(272.601097780684,91.9144533088616,272.32368984116));
#20681=CARTESIAN_POINT('Ctrl Pts',(272.556053140956,91.912897347606,272.350402646128));
#20682=CARTESIAN_POINT('Ctrl Pts',(272.510574130833,91.91119309357,272.376196962215));
#20683=CARTESIAN_POINT('Ctrl Pts',(272.472354806289,91.909760884779,272.397873804681));
#20684=CARTESIAN_POINT('Ctrl Pts',(272.433827432696,91.9082239447931,272.418901728127));
#20685=CARTESIAN_POINT('Ctrl Pts',(272.395144319412,91.906580460314,272.439340662118));
#20686=CARTESIAN_POINT('Ctrl Pts',(272.336857160485,91.9041040815303,272.470137753995));
#20687=CARTESIAN_POINT('Ctrl Pts',(272.278033409372,91.9013833209367,272.499695719002));
#20688=CARTESIAN_POINT('Ctrl Pts',(272.218759135935,91.8984096788626,272.528225589475));
#20689=CARTESIAN_POINT('Ctrl Pts',(272.155384374984,91.8952303255837,272.55872910502));
#20690=CARTESIAN_POINT('Ctrl Pts',(272.091494349814,91.8917620135632,272.588057263861));
#20691=CARTESIAN_POINT('Ctrl Pts',(272.027142805416,91.8879897181143,272.616435627212));
#20692=CARTESIAN_POINT('Ctrl Pts',(271.991734012766,91.8859140503332,272.632050537359));
#20693=CARTESIAN_POINT('Ctrl Pts',(271.956184629353,91.8837462565477,272.647377337366));
#20694=CARTESIAN_POINT('Ctrl Pts',(271.920498131808,91.8814830897533,272.662450052827));
#20695=CARTESIAN_POINT('Ctrl Pts',(271.862268990929,91.8777903132925,272.687043984212));
#20696=CARTESIAN_POINT('Ctrl Pts',(271.803630523397,91.8738384340663,272.71096347216));
#20697=CARTESIAN_POINT('Ctrl Pts',(271.744674380866,91.8696265270691,272.734262818706));
#20698=CARTESIAN_POINT('Ctrl Pts',(271.650842289134,91.8629230348331,272.771345068808));
#20699=CARTESIAN_POINT('Ctrl Pts',(271.556130751135,91.8555536840876,272.806886942222));
#20700=CARTESIAN_POINT('Ctrl Pts',(271.461255325209,91.8475267985236,272.840905168818));
#20701=CARTESIAN_POINT('Ctrl Pts',(271.445179827524,91.8461667394879,272.846669147399));
#20702=CARTESIAN_POINT('Ctrl Pts',(271.429099510396,91.8447877834954,272.852389348935));
#20703=CARTESIAN_POINT('Ctrl Pts',(271.413017727445,91.8433899471151,272.858065811931));
#20704=CARTESIAN_POINT('Ctrl Pts',(271.293504536816,91.8330018025733,272.900250948124));
#20705=CARTESIAN_POINT('Ctrl Pts',(271.173507435133,91.8215530737852,272.940190217739));
#20706=CARTESIAN_POINT('Ctrl Pts',(271.052959917239,91.8089715978704,272.978194428691));
#20707=CARTESIAN_POINT('Ctrl Pts',(270.999522572895,91.8033943726187,272.995041263389));
#20708=CARTESIAN_POINT('Ctrl Pts',(270.945976758625,91.7975942994658,273.011507245252));
#20709=CARTESIAN_POINT('Ctrl Pts',(270.892315466622,91.7915637910068,273.027616795162));
#20710=CARTESIAN_POINT('Ctrl Pts',(270.860374894621,91.7879742782976,273.037205610854));
#20711=CARTESIAN_POINT('Ctrl Pts',(270.828394131352,91.7843034378172,273.046670107705));
#20712=CARTESIAN_POINT('Ctrl Pts',(270.796369186396,91.7805492689741,273.056012079442));
#20713=CARTESIAN_POINT('Ctrl Pts',(270.521104434134,91.7482809744325,273.136309345819));
#20714=CARTESIAN_POINT('Ctrl Pts',(270.243771310296,91.7099651949295,273.207231978851));
#20715=CARTESIAN_POINT('Ctrl Pts',(269.965387262019,91.6648266164728,273.269078101933));
#20716=CARTESIAN_POINT('Ctrl Pts',(269.920224430833,91.6575036897053,273.279111528897));
#20717=CARTESIAN_POINT('Ctrl Pts',(269.875033852327,91.6500012300741,273.28890601228));
#20718=CARTESIAN_POINT('Ctrl Pts',(269.82981977108,91.6423159687712,273.29846276181));
#20719=CARTESIAN_POINT('Ctrl Pts',(274.135356630693,91.9232791773928,271.539778446323));
#20720=CARTESIAN_POINT('Ctrl Pts',(273.694940779298,91.8262033907668,271.539778446323));
#20721=CARTESIAN_POINT('Ctrl Pts',(273.255484225105,91.9275333837837,271.539778446323));
#20722=CARTESIAN_POINT('Ctrl Pts',(274.135356618139,91.9232791746256,271.77352759202));
#20723=CARTESIAN_POINT('Ctrl Pts',(273.694940766237,91.8262033874431,271.712138594175));
#20724=CARTESIAN_POINT('Ctrl Pts',(273.255484212108,91.9275333867805,271.656653018791));
#20725=CARTESIAN_POINT('Ctrl Pts',(274.094104920322,91.9143299491368,272.001710787058));
#20726=CARTESIAN_POINT('Ctrl Pts',(273.651729880129,91.8153819562333,271.880756949373));
#20727=CARTESIAN_POINT('Ctrl Pts',(273.210441477653,91.927321339897,271.77074461716));
#20728=CARTESIAN_POINT('Ctrl Pts',(273.948712475437,91.8809612331079,272.43610810231));
#20729=CARTESIAN_POINT('Ctrl Pts',(273.500699311358,91.7755432830053,272.197958934196));
#20730=CARTESIAN_POINT('Ctrl Pts',(273.051917078416,91.9254721937242,271.987943273847));
#20731=CARTESIAN_POINT('Ctrl Pts',(273.848753385412,91.8573753781329,272.634456464127));
#20732=CARTESIAN_POINT('Ctrl Pts',(273.396675272924,91.7473695895106,272.341448843629));
#20733=CARTESIAN_POINT('Ctrl Pts',(272.943010608921,91.9238122517172,272.087117455614));
#20734=CARTESIAN_POINT('Ctrl Pts',(273.61549231008,91.7983990370043,273.007566223003));
#20735=CARTESIAN_POINT('Ctrl Pts',(273.155975276006,91.6778806512037,272.606580240907));
#20736=CARTESIAN_POINT('Ctrl Pts',(272.689365096497,91.9175643010313,272.273672334273));
#20737=CARTESIAN_POINT('Ctrl Pts',(273.48331851805,91.7632558189231,273.179638632332));
#20738=CARTESIAN_POINT('Ctrl Pts',(273.019825191783,91.636639842145,272.726492502695));
#20739=CARTESIAN_POINT('Ctrl Pts',(272.545857611411,91.9129836201679,272.359708539774));
#20740=CARTESIAN_POINT('Ctrl Pts',(273.205089743305,91.6840327233082,273.498166259421));
#20741=CARTESIAN_POINT('Ctrl Pts',(272.735652702075,91.5449382008264,272.94309386566));
#20742=CARTESIAN_POINT('Ctrl Pts',(272.244430498303,91.9001776457436,272.518972352425));
#20743=CARTESIAN_POINT('Ctrl Pts',(273.057913590941,91.6396897520155,273.645915370351));
#20744=CARTESIAN_POINT('Ctrl Pts',(272.58594546409,91.4939300491432,273.040692149937));
#20745=CARTESIAN_POINT('Ctrl Pts',(272.085289161225,91.8919346167594,272.592846908584));
#20746=CARTESIAN_POINT('Ctrl Pts',(272.752379380603,91.5413516256883,273.924324537817));
#20747=CARTESIAN_POINT('Ctrl Pts',(272.27815788873,91.3824825706594,273.218316332999));
#20748=CARTESIAN_POINT('Ctrl Pts',(271.755705227879,91.8710331819526,272.732051491823));
#20749=CARTESIAN_POINT('Ctrl Pts',(272.593678387909,91.4872118120189,274.055012603804));
#20750=CARTESIAN_POINT('Ctrl Pts',(272.119348482168,91.321650261883,273.298198175737));
#20751=CARTESIAN_POINT('Ctrl Pts',(271.584897011395,91.8583306460472,272.797395525323));
#20752=CARTESIAN_POINT('Ctrl Pts',(272.273457666484,91.3709349540835,274.297680104029));
#20753=CARTESIAN_POINT('Ctrl Pts',(271.80251742236,91.1931416236028,273.439263812478));
#20754=CARTESIAN_POINT('Ctrl Pts',(271.241131095768,91.8284570802143,272.918729274917));
#20755=CARTESIAN_POINT('Ctrl Pts',(272.111164141465,91.3085699747133,274.410345911472));
#20756=CARTESIAN_POINT('Ctrl Pts',(271.64342889865,91.1249694608679,273.500705767743));
#20757=CARTESIAN_POINT('Ctrl Pts',(271.067336037362,91.8112458522357,272.975062179002));
#20758=CARTESIAN_POINT('Ctrl Pts',(271.619489127284,91.1082362789725,274.725628850557));
#20759=CARTESIAN_POINT('Ctrl Pts',(271.163441768428,90.9080618135687,273.661531752826));
#20760=CARTESIAN_POINT('Ctrl Pts',(270.542249033313,91.7522310661092,273.13270364823));
#20761=CARTESIAN_POINT('Ctrl Pts',(271.285463185231,90.9571441468218,274.905982351229));
#20762=CARTESIAN_POINT('Ctrl Pts',(270.847729939072,90.7494407701335,273.733052553961));
#20763=CARTESIAN_POINT('Ctrl Pts',(270.187343357388,91.7030860232968,273.222894193987));
#20764=CARTESIAN_POINT('Ctrl Pts',(270.946701599761,90.7857513677001,275.057147077298));
#20765=CARTESIAN_POINT('Ctrl Pts',(270.548229297884,90.5841485940949,273.76942958616));
#20766=CARTESIAN_POINT('Ctrl Pts',(269.82981977108,91.6423159687712,273.29846276181));
#20767=CARTESIAN_POINT('Origin',(273.70485351704,93.8763964470762,271.539778446323));
#20768=CARTESIAN_POINT('Origin',(289.522998818702,72.7829756068832,232.288983442877));
#20769=CARTESIAN_POINT('Origin',(259.80186267196,79.6360819935406,232.288983442877));
#20770=CARTESIAN_POINT('Origin',(273.70485351704,93.8763964470762,225.073593133703));
#20771=CARTESIAN_POINT('Origin',(273.70485351704,93.8763964470762,234.607407821084));
#20772=CARTESIAN_POINT('Origin',(292.443899216281,85.4505855182842,234.607407821084));
#20773=CARTESIAN_POINT('Ctrl Pts',(269.82981977108,91.6423159687712,232.848723505596));
#20774=CARTESIAN_POINT('Ctrl Pts',(270.015561437251,91.6738873996182,232.887983101985));
#20775=CARTESIAN_POINT('Ctrl Pts',(270.200459723154,91.7023018694398,232.93115673308));
#20776=CARTESIAN_POINT('Ctrl Pts',(270.384451598149,91.7278499278192,232.978338693559));
#20777=CARTESIAN_POINT('Ctrl Pts',(270.521635861377,91.7468985492097,233.013517543094));
#20778=CARTESIAN_POINT('Ctrl Pts',(270.65831599323,91.7643530228057,233.050925525407));
#20779=CARTESIAN_POINT('Ctrl Pts',(270.794458168282,91.7803254248894,233.090616791577));
#20780=CARTESIAN_POINT('Ctrl Pts',(270.827503889548,91.7842023979656,233.100251032532));
#20781=CARTESIAN_POINT('Ctrl Pts',(270.860514172686,91.7879920027267,233.110019115394));
#20782=CARTESIAN_POINT('Ctrl Pts',(270.893491220388,91.7916960151221,233.119922617088));
#20783=CARTESIAN_POINT('Ctrl Pts',(271.019946239265,91.8058995594058,233.157898954599));
#20784=CARTESIAN_POINT('Ctrl Pts',(271.145979477639,91.818840099349,233.197817538844));
#20785=CARTESIAN_POINT('Ctrl Pts',(271.271436525776,91.8305893739001,233.240086590348));
#20786=CARTESIAN_POINT('Ctrl Pts',(271.387350430509,91.8414449161849,233.279140361196));
#20787=CARTESIAN_POINT('Ctrl Pts',(271.502772822986,91.8512832807417,233.320200439574));
#20788=CARTESIAN_POINT('Ctrl Pts',(271.617555868356,91.860152164324,233.363624493924));
#20789=CARTESIAN_POINT('Ctrl Pts',(271.658627289105,91.8633256090432,233.379162395023));
#20790=CARTESIAN_POINT('Ctrl Pts',(271.69961657089,91.8663748568654,233.395003328621));
#20791=CARTESIAN_POINT('Ctrl Pts',(271.740515912666,91.8693018708402,233.411164981821));
#20792=CARTESIAN_POINT('Ctrl Pts',(271.799838261565,91.8735473510047,233.434606611642));
#20793=CARTESIAN_POINT('Ctrl Pts',(271.858885216673,91.8775346062734,233.458693452383));
#20794=CARTESIAN_POINT('Ctrl Pts',(271.917789704208,91.8812783618145,233.483545832084));
#20795=CARTESIAN_POINT('Ctrl Pts',(271.98067891853,91.8852753721348,233.510079407009));
#20796=CARTESIAN_POINT('Ctrl Pts',(272.043187679696,91.8889798656512,233.537425061905));
#20797=CARTESIAN_POINT('Ctrl Pts',(272.105263898368,91.8924068510043,233.565755425312));
#20798=CARTESIAN_POINT('Ctrl Pts',(272.162046353164,91.8955415883492,233.591669819165));
#20799=CARTESIAN_POINT('Ctrl Pts',(272.218467233987,91.8984440130497,233.618408205897));
#20800=CARTESIAN_POINT('Ctrl Pts',(272.274449019999,91.9011207122047,233.646122140915));
#20801=CARTESIAN_POINT('Ctrl Pts',(272.315013893718,91.9030602709602,233.666203891684));
#20802=CARTESIAN_POINT('Ctrl Pts',(272.355347522225,91.9048812121483,233.686798232757));
#20803=CARTESIAN_POINT('Ctrl Pts',(272.395404653415,91.9065846709651,233.707969914034));
#20804=CARTESIAN_POINT('Ctrl Pts',(272.439578572256,91.9084631991894,233.731317470453));
#20805=CARTESIAN_POINT('Ctrl Pts',(272.483534972761,91.9102014129653,233.755434280492));
#20806=CARTESIAN_POINT('Ctrl Pts',(272.527036273113,91.9118021664447,233.78039055539));
#20807=CARTESIAN_POINT('Ctrl Pts',(272.566794344995,91.9132651772372,233.80319937635));
#20808=CARTESIAN_POINT('Ctrl Pts',(272.60617228052,91.9146133414286,233.826709489539));
#20809=CARTESIAN_POINT('Ctrl Pts',(272.644950932319,91.9158481686079,233.850980212717));
#20810=CARTESIAN_POINT('Ctrl Pts',(272.677190170571,91.9168747614827,233.871158057762));
#20811=CARTESIAN_POINT('Ctrl Pts',(272.708956236063,91.9178216757778,233.891824193169));
#20812=CARTESIAN_POINT('Ctrl Pts',(272.740208285718,91.9186928087398,233.913085540272));
#20813=CARTESIAN_POINT('Ctrl Pts',(272.766064785827,91.9194135438524,233.930676195277));
#20814=CARTESIAN_POINT('Ctrl Pts',(272.791569024412,91.9200823513293,233.94867448331));
#20815=CARTESIAN_POINT('Ctrl Pts',(272.816671412602,91.9207001828372,233.967147124109));
#20816=CARTESIAN_POINT('Ctrl Pts',(272.843301300097,91.9213556098597,233.986743839071));
#20817=CARTESIAN_POINT('Ctrl Pts',(272.869552519657,91.9219560900281,234.006908595747));
#20818=CARTESIAN_POINT('Ctrl Pts',(272.895300543815,91.9225047161967,234.027756395878));
#20819=CARTESIAN_POINT('Ctrl Pts',(272.920502151311,91.9230416995891,234.048161770398));
#20820=CARTESIAN_POINT('Ctrl Pts',(272.945222322143,91.9235289788969,234.069221401029));
#20821=CARTESIAN_POINT('Ctrl Pts',(272.969294562453,91.9239691023271,234.091056293083));
#20822=CARTESIAN_POINT('Ctrl Pts',(272.991562003493,91.924376227813,234.111254129478));
#20823=CARTESIAN_POINT('Ctrl Pts',(273.013275095638,91.9247429811296,234.132115361817));
#20824=CARTESIAN_POINT('Ctrl Pts',(273.034255030787,91.9250714239154,234.153747492021));
#20825=CARTESIAN_POINT('Ctrl Pts',(273.035955476365,91.925098044545,234.155500798687));
#20826=CARTESIAN_POINT('Ctrl Pts',(273.037651077778,91.9251244136322,234.157259176335));
#20827=CARTESIAN_POINT('Ctrl Pts',(273.039341724696,91.9251505323558,234.159022685846));
#20828=CARTESIAN_POINT('Ctrl Pts',(273.058417945833,91.9254452399859,234.17892104371));
#20829=CARTESIAN_POINT('Ctrl Pts',(273.076927481094,91.9257089467546,234.199534667638));
#20830=CARTESIAN_POINT('Ctrl Pts',(273.094667580603,91.9259425960946,234.220959767754));
#20831=CARTESIAN_POINT('Ctrl Pts',(273.107225770739,91.9261079961159,234.236126564354));
#20832=CARTESIAN_POINT('Ctrl Pts',(273.11939749702,91.9262583450989,234.251700218268));
#20833=CARTESIAN_POINT('Ctrl Pts',(273.131095302992,91.9263942221247,234.267718436237));
#20834=CARTESIAN_POINT('Ctrl Pts',(273.146911991866,91.9265779424434,234.289376785718));
#20835=CARTESIAN_POINT('Ctrl Pts',(273.16170916562,91.9267367413741,234.31169009652));
#20836=CARTESIAN_POINT('Ctrl Pts',(273.175229567178,91.9268714448707,234.334711651649));
#20837=CARTESIAN_POINT('Ctrl Pts',(273.180570546791,91.9269246569463,234.343805882769));
#20838=CARTESIAN_POINT('Ctrl Pts',(273.185711732346,91.9269741156589,234.353010655731));
#20839=CARTESIAN_POINT('Ctrl Pts',(273.190634985725,91.9270199005296,234.362329333268));
#20840=CARTESIAN_POINT('Ctrl Pts',(273.200954484681,91.9271158689653,234.381861962547));
#20841=CARTESIAN_POINT('Ctrl Pts',(273.210366129408,91.9271982025984,234.402014498081));
#20842=CARTESIAN_POINT('Ctrl Pts',(273.218596491308,91.9272662961898,234.422661527238));
#20843=CARTESIAN_POINT('Ctrl Pts',(273.22647599308,91.9273314869531,234.442428374046));
#20844=CARTESIAN_POINT('Ctrl Pts',(273.233272329597,91.9273836561975,234.462648391072));
#20845=CARTESIAN_POINT('Ctrl Pts',(273.238790086692,91.9274236510184,234.483204447906));
#20846=CARTESIAN_POINT('Ctrl Pts',(273.244214637016,91.9274629702408,234.503413268778));
#20847=CARTESIAN_POINT('Ctrl Pts',(273.248402941013,91.92749054973,234.523946829525));
#20848=CARTESIAN_POINT('Ctrl Pts',(273.251220475383,91.9275081462254,234.544687559797));
#20849=CARTESIAN_POINT('Ctrl Pts',(273.254038009754,91.9275257427209,234.56542829007));
#20850=CARTESIAN_POINT('Ctrl Pts',(273.255484226474,91.927533383468,234.586376152881));
#20851=CARTESIAN_POINT('Ctrl Pts',(273.255484225105,91.9275333837837,234.607407821084));
#20852=CARTESIAN_POINT('Ctrl Pts',(259.737667058827,79.3576729844988,230.309496805655));
#20853=CARTESIAN_POINT('Ctrl Pts',(259.352493380025,77.6872189302482,230.556932635308));
#20854=CARTESIAN_POINT('Ctrl Pts',(259.352493380025,77.6872189302482,232.288983442877));
#20855=CARTESIAN_POINT('Ctrl Pts',(260.489866638734,79.1842306313197,230.309496805879));
#20856=CARTESIAN_POINT('Ctrl Pts',(259.96963870844,77.5449174176977,230.556932635576));
#20857=CARTESIAN_POINT('Ctrl Pts',(259.950395610518,77.5493544968644,232.288983443048));
#20858=CARTESIAN_POINT('Ctrl Pts',(261.204913401151,78.9177192700331,230.32315997602));
#20859=CARTESIAN_POINT('Ctrl Pts',(260.556326304222,77.3317737998227,230.575081299956));
#20860=CARTESIAN_POINT('Ctrl Pts',(260.520304163103,77.3441824757216,232.301458511035));
#20861=CARTESIAN_POINT('Ctrl Pts',(262.223292632623,78.383567916756,230.369110269103));
#20862=CARTESIAN_POINT('Ctrl Pts',(261.399847181909,76.9039004839053,230.632620004888));
#20863=CARTESIAN_POINT('Ctrl Pts',(261.334314889639,76.9392458488658,232.343413127113));
#20864=CARTESIAN_POINT('Ctrl Pts',(262.555366780788,78.1816425648538,230.38896060812));
#20865=CARTESIAN_POINT('Ctrl Pts',(261.6753798258,76.742552789912,230.657062473388));
#20866=CARTESIAN_POINT('Ctrl Pts',(261.600168265845,76.7869681618154,232.361537349181));
#20867=CARTESIAN_POINT('Ctrl Pts',(263.192272886508,77.7364025768308,230.439567449033));
#20868=CARTESIAN_POINT('Ctrl Pts',(262.205789159917,76.3857612367115,230.717576280988));
#20869=CARTESIAN_POINT('Ctrl Pts',(262.110942369255,76.4526422432372,232.407743595821));
#20870=CARTESIAN_POINT('Ctrl Pts',(263.494777280234,77.4950731950091,230.470081140236));
#20871=CARTESIAN_POINT('Ctrl Pts',(262.458640311379,76.1920833314033,230.753306404236));
#20872=CARTESIAN_POINT('Ctrl Pts',(262.353991061074,76.2720769658325,232.435603921899));
#20873=CARTESIAN_POINT('Ctrl Pts',(264.068873292152,76.9765864414354,230.544184477118));
#20874=CARTESIAN_POINT('Ctrl Pts',(262.93982714268,75.7742357891063,230.837564148899));
#20875=CARTESIAN_POINT('Ctrl Pts',(262.816166800432,75.8852869421232,232.503263491111));
#20876=CARTESIAN_POINT('Ctrl Pts',(264.340460862299,76.6994232039253,230.587767815121));
#20877=CARTESIAN_POINT('Ctrl Pts',(263.168240525539,75.5501498442423,230.886047592305));
#20878=CARTESIAN_POINT('Ctrl Pts',(263.035290733391,75.6790579795884,232.543056972796));
#20879=CARTESIAN_POINT('Ctrl Pts',(264.852462244799,76.109492954915,230.691718673468));
#20880=CARTESIAN_POINT('Ctrl Pts',(263.599273270706,75.0709585050467,230.998556574986));
#20881=CARTESIAN_POINT('Ctrl Pts',(263.449407025873,75.2411080436715,232.637968626996));
#20882=CARTESIAN_POINT('Ctrl Pts',(265.094373229635,75.7942915062606,230.752634143475));
#20883=CARTESIAN_POINT('Ctrl Pts',(263.803351197743,74.8137915708696,231.063135696844));
#20884=CARTESIAN_POINT('Ctrl Pts',(263.645621061591,75.0075891196608,232.693587098739));
#20885=CARTESIAN_POINT('Ctrl Pts',(265.756639414064,74.8164649195093,230.963024899036));
#20886=CARTESIAN_POINT('Ctrl Pts',(264.360159533119,74.0132571206067,231.280658468406));
#20887=CARTESIAN_POINT('Ctrl Pts',(264.18452429865,74.2844949805711,232.885683007215));
#20888=CARTESIAN_POINT('Ctrl Pts',(266.116520847411,74.1216801997293,231.139458375964));
#20889=CARTESIAN_POINT('Ctrl Pts',(264.662785788949,73.4369654879794,231.457867253309));
#20890=CARTESIAN_POINT('Ctrl Pts',(264.479839828954,73.7723884511474,233.046772261445));
#20891=CARTESIAN_POINT('Ctrl Pts',(266.39885077907,73.3906559987533,231.366755111123));
#20892=CARTESIAN_POINT('Ctrl Pts',(264.891797790303,72.8283445041923,231.677295442204));
#20893=CARTESIAN_POINT('Ctrl Pts',(264.714335805196,73.2350168556771,233.254306243521));
#20894=CARTESIAN_POINT('Ctrl Pts',(264.697446445794,73.2734364402351,233.239531476064));
#20895=CARTESIAN_POINT('Ctrl Pts',(264.654229186946,73.3710281088638,233.167817844006));
#20896=CARTESIAN_POINT('Ctrl Pts',(264.609313044049,73.4689055458569,233.096787663571));
#20897=CARTESIAN_POINT('Ctrl Pts',(264.562879524106,73.5667785698821,233.026632701688));
#20898=CARTESIAN_POINT('Ctrl Pts',(264.516195848542,73.665178874352,232.956099787454));
#20899=CARTESIAN_POINT('Ctrl Pts',(264.467978434442,73.7635743807309,232.88645157777));
#20900=CARTESIAN_POINT('Ctrl Pts',(264.418450588595,73.8616684422313,232.817847262986));
#20901=CARTESIAN_POINT('Ctrl Pts',(264.40679314368,73.884756991691,232.801699760366));
#20902=CARTESIAN_POINT('Ctrl Pts',(264.395063267842,73.9078288468005,232.78560993391));
#20903=CARTESIAN_POINT('Ctrl Pts',(264.383264177312,73.9308801593125,232.769579574183));
#20904=CARTESIAN_POINT('Ctrl Pts',(264.313305252971,74.0675555262783,232.674532695741));
#20905=CARTESIAN_POINT('Ctrl Pts',(264.240690520829,74.2039410093792,232.581287471137));
#20906=CARTESIAN_POINT('Ctrl Pts',(264.165615557534,74.3400654072201,232.489700248591));
#20907=CARTESIAN_POINT('Ctrl Pts',(264.120725662995,74.4214588517848,232.434937108116));
#20908=CARTESIAN_POINT('Ctrl Pts',(264.074956495285,74.5027582590142,232.380767208533));
#20909=CARTESIAN_POINT('Ctrl Pts',(264.028354597553,74.5839630677654,232.327163638241));
#20910=CARTESIAN_POINT('Ctrl Pts',(263.985456304859,74.6587142651096,232.277820118777));
#20911=CARTESIAN_POINT('Ctrl Pts',(263.941868682874,74.7333559521437,232.228977938585));
#20912=CARTESIAN_POINT('Ctrl Pts',(263.897622680722,74.8078999837302,232.180607335982));
#20913=CARTESIAN_POINT('Ctrl Pts',(263.825507862472,74.9293963682165,232.101769993722));
#20914=CARTESIAN_POINT('Ctrl Pts',(263.751669999091,75.0506924616519,232.024180793303));
#20915=CARTESIAN_POINT('Ctrl Pts',(263.676293153804,75.1720265572414,231.947761794839));
#20916=CARTESIAN_POINT('Ctrl Pts',(263.603251188336,75.2896021971659,231.873709958022));
#20917=CARTESIAN_POINT('Ctrl Pts',(263.528763284777,75.4072132185362,231.800757130054));
#20918=CARTESIAN_POINT('Ctrl Pts',(263.453038257345,75.5250695290885,231.728853068671));
#20919=CARTESIAN_POINT('Ctrl Pts',(263.394019028683,75.6169254026021,231.672811857669));
#20920=CARTESIAN_POINT('Ctrl Pts',(263.334291283429,75.7088649691641,231.617453519133));
#20921=CARTESIAN_POINT('Ctrl Pts',(263.274112511905,75.8008447270264,231.562900942566));
#20922=CARTESIAN_POINT('Ctrl Pts',(263.256213869813,75.8282017621411,231.546675668795));
#20923=CARTESIAN_POINT('Ctrl Pts',(263.238275603622,75.8555622284378,231.530521839858));
#20924=CARTESIAN_POINT('Ctrl Pts',(263.22030522037,75.8829246557764,231.51444312478));
#20925=CARTESIAN_POINT('Ctrl Pts',(263.165709508658,75.9660542793201,231.465594478605));
#20926=CARTESIAN_POINT('Ctrl Pts',(263.110705657456,76.0493669964364,231.417342430414));
#20927=CARTESIAN_POINT('Ctrl Pts',(263.055520334322,76.1328170019997,231.369809600742));
#20928=CARTESIAN_POINT('Ctrl Pts',(263.038785104679,76.158123640205,231.355395028625));
#20929=CARTESIAN_POINT('Ctrl Pts',(263.022033475043,76.1834427777927,231.341046764967));
#20930=CARTESIAN_POINT('Ctrl Pts',(263.005272555421,76.2087727973911,231.326768677458));
#20931=CARTESIAN_POINT('Ctrl Pts',(262.947061992686,76.2967437875341,231.277180974194));
#20932=CARTESIAN_POINT('Ctrl Pts',(262.888651064932,76.384974810687,231.228304565985));
#20933=CARTESIAN_POINT('Ctrl Pts',(262.830207117975,76.4736562503305,231.180271844975));
#20934=CARTESIAN_POINT('Ctrl Pts',(262.773496656583,76.5597073406654,231.133663805781));
#20935=CARTESIAN_POINT('Ctrl Pts',(262.716754900792,76.646182300906,231.087850087869));
#20936=CARTESIAN_POINT('Ctrl Pts',(262.660170090237,76.7332741961984,231.042976730252));
#20937=CARTESIAN_POINT('Ctrl Pts',(262.606111579047,76.8164777653204,231.000106799592));
#20938=CARTESIAN_POINT('Ctrl Pts',(262.552196231045,76.9002442747484,230.958095150216));
#20939=CARTESIAN_POINT('Ctrl Pts',(262.498622814573,76.9847622690485,230.917092579518));
#20940=CARTESIAN_POINT('Ctrl Pts',(262.451137883189,77.0596750042147,230.880749848657));
#20941=CARTESIAN_POINT('Ctrl Pts',(262.403921887061,77.1351782564116,230.845200112458));
#20942=CARTESIAN_POINT('Ctrl Pts',(262.357138788268,77.2114190794966,230.810565027849));
#20943=CARTESIAN_POINT('Ctrl Pts',(262.31561657369,77.2790864187155,230.779824750864));
#20944=CARTESIAN_POINT('Ctrl Pts',(262.274464121646,77.3472811150659,230.749829012529));
#20945=CARTESIAN_POINT('Ctrl Pts',(262.233715133929,77.4162867755718,230.720601932399));
#20946=CARTESIAN_POINT('Ctrl Pts',(262.219591643633,77.4402039531783,230.710471904496));
#20947=CARTESIAN_POINT('Ctrl Pts',(262.205516943508,77.4642186345719,230.700434512941));
#20948=CARTESIAN_POINT('Ctrl Pts',(262.191493523411,77.4883429401725,230.690491742317));
#20949=CARTESIAN_POINT('Ctrl Pts',(262.153645195841,77.5534529215029,230.663656830653));
#20950=CARTESIAN_POINT('Ctrl Pts',(262.116452720228,77.6188974008809,230.637693868061));
#20951=CARTESIAN_POINT('Ctrl Pts',(262.079950203966,77.6848975804388,230.612712308445));
#20952=CARTESIAN_POINT('Ctrl Pts',(262.044800464362,77.7484518052682,230.588656560914));
#20953=CARTESIAN_POINT('Ctrl Pts',(262.010290480822,77.8125210117592,230.565510694921));
#20954=CARTESIAN_POINT('Ctrl Pts',(261.976479795831,77.8773102687136,230.543410702692));
#20955=CARTESIAN_POINT('Ctrl Pts',(261.968393922972,77.8928047106185,230.538125458474));
#20956=CARTESIAN_POINT('Ctrl Pts',(261.960348181157,77.9083403809965,230.532900214237));
#20957=CARTESIAN_POINT('Ctrl Pts',(261.952343646247,77.9239201814014,230.527737185114));
#20958=CARTESIAN_POINT('Ctrl Pts',(261.915421006234,77.9957853638597,230.503921602098));
#20959=CARTESIAN_POINT('Ctrl Pts',(261.879415499712,78.0685007726458,230.48145621462));
#20960=CARTESIAN_POINT('Ctrl Pts',(261.844512219108,78.1422191631716,230.460620223486));
#20961=CARTESIAN_POINT('Ctrl Pts',(261.810342116173,78.2143890265434,230.440221912798));
#20962=CARTESIAN_POINT('Ctrl Pts',(261.777228382095,78.2875199945043,230.421385152265));
#20963=CARTESIAN_POINT('Ctrl Pts',(261.745364910435,78.3617834768448,230.404406843503));
#20964=CARTESIAN_POINT('Ctrl Pts',(261.714466316366,78.4337981405152,230.387942665463));
#20965=CARTESIAN_POINT('Ctrl Pts',(261.684743410344,78.506877645955,230.373226044139));
#20966=CARTESIAN_POINT('Ctrl Pts',(261.656392439806,78.5812071226677,230.360561957802));
#20967=CARTESIAN_POINT('Ctrl Pts',(261.641714198808,78.6196899665266,230.35400533883));
#20968=CARTESIAN_POINT('Ctrl Pts',(261.627404024125,78.658508350682,230.347999468436));
#20969=CARTESIAN_POINT('Ctrl Pts',(261.613491303169,78.6976913251228,230.342590522453));
#20970=CARTESIAN_POINT('Ctrl Pts',(270.946701599761,90.7857513677001,231.090039190109));
#20971=CARTESIAN_POINT('Ctrl Pts',(270.548229297884,90.584148594095,232.377756681246));
#20972=CARTESIAN_POINT('Ctrl Pts',(269.82981977108,91.6423159687712,232.848723505596));
#20973=CARTESIAN_POINT('Ctrl Pts',(271.286862403972,90.9578520664885,231.241828286301));
#20974=CARTESIAN_POINT('Ctrl Pts',(270.848946691457,90.7501122866934,232.414281499181));
#20975=CARTESIAN_POINT('Ctrl Pts',(270.188821842695,91.7033373287686,232.924604575929));
#20976=CARTESIAN_POINT('Ctrl Pts',(271.6212194979,91.1089748570485,231.422589429823));
#20977=CARTESIAN_POINT('Ctrl Pts',(271.165120845064,90.9088548773701,232.486141144197));
#20978=CARTESIAN_POINT('Ctrl Pts',(270.544092776974,91.752458983209,233.01499862562));
#20979=CARTESIAN_POINT('Ctrl Pts',(272.275527462515,91.375506398507,231.842314946566));
#20980=CARTESIAN_POINT('Ctrl Pts',(271.798039921684,91.1948055159721,232.698358378032));
#20981=CARTESIAN_POINT('Ctrl Pts',(271.24287296878,91.830953766497,233.224861383659));
#20982=CARTESIAN_POINT('Ctrl Pts',(272.595862729514,91.4909084601913,232.080552096927));
#20983=CARTESIAN_POINT('Ctrl Pts',(272.117008863945,91.3240589446257,232.836133673852));
#20984=CARTESIAN_POINT('Ctrl Pts',(271.586877031609,91.8602853819312,233.343979959847));
#20985=CARTESIAN_POINT('Ctrl Pts',(273.055973002656,91.6390983881989,232.499348715414));
#20986=CARTESIAN_POINT('Ctrl Pts',(272.583967923736,91.4932491614987,233.105225965723));
#20987=CARTESIAN_POINT('Ctrl Pts',(272.083191646016,91.891821899915,233.553378267828));
#20988=CARTESIAN_POINT('Ctrl Pts',(273.204529404127,91.6838758628784,232.648354966299));
#20989=CARTESIAN_POINT('Ctrl Pts',(272.735069316385,91.5447528864996,233.203629145364));
#20990=CARTESIAN_POINT('Ctrl Pts',(272.243823100579,91.9001534779783,233.627881394136));
#20991=CARTESIAN_POINT('Ctrl Pts',(273.484341261294,91.7635443402254,232.968742094674));
#20992=CARTESIAN_POINT('Ctrl Pts',(273.020860725553,91.6369710951425,233.421501455589));
#20993=CARTESIAN_POINT('Ctrl Pts',(272.546965968386,91.9130290682149,233.788074957434));
#20994=CARTESIAN_POINT('Ctrl Pts',(273.616857737478,91.7987484382474,233.141703545685));
#20995=CARTESIAN_POINT('Ctrl Pts',(273.15739221448,91.6782943342807,233.542090459735));
#20996=CARTESIAN_POINT('Ctrl Pts',(272.690849322385,91.9176033917613,233.874555683821));
#20997=CARTESIAN_POINT('Ctrl Pts',(273.848277352538,91.8572508300294,233.512069308584));
#20998=CARTESIAN_POINT('Ctrl Pts',(273.396194529834,91.7472262082025,233.805283770732));
#20999=CARTESIAN_POINT('Ctrl Pts',(272.942493502819,91.9237969739132,234.059738564397));
#21000=CARTESIAN_POINT('Ctrl Pts',(273.948668648815,91.8809506992841,233.711024516524));
#21001=CARTESIAN_POINT('Ctrl Pts',(273.500654142745,91.77553083905,233.949189921464));
#21002=CARTESIAN_POINT('Ctrl Pts',(273.051869353513,91.9254713513345,234.159216168977));
#21003=CARTESIAN_POINT('Ctrl Pts',(274.09398531746,91.9143029740673,234.145040928275));
#21004=CARTESIAN_POINT('Ctrl Pts',(273.651605727385,91.8153497331837,234.266111504467));
#21005=CARTESIAN_POINT('Ctrl Pts',(273.210311012066,91.9273201034252,234.376224374506));
#21006=CARTESIAN_POINT('Ctrl Pts',(274.135356638104,91.9232791790263,234.372165957108));
#21007=CARTESIAN_POINT('Ctrl Pts',(273.694940786991,91.8262033927225,234.433947592198));
#21008=CARTESIAN_POINT('Ctrl Pts',(273.255484232762,91.9275333820181,234.489786889222));
#21009=CARTESIAN_POINT('Ctrl Pts',(274.135356630693,91.9232791773928,234.607407821084));
#21010=CARTESIAN_POINT('Ctrl Pts',(273.694940779299,91.8262033907668,234.607407821084));
#21011=CARTESIAN_POINT('Ctrl Pts',(273.255484225105,91.9275333837837,234.607407821084));
#21012=CARTESIAN_POINT('Origin',(270.043805148192,92.5703459989105,231.090039190109));
#21013=CARTESIAN_POINT('Ctrl Pts',(261.613491303076,78.6976913253861,230.342590522417));
#21014=CARTESIAN_POINT('Ctrl Pts',(263.538250261041,78.7291375341272,230.271134115559));
#21015=CARTESIAN_POINT('Ctrl Pts',(263.544486310321,78.4442745295379,228.365981599697));
#21016=CARTESIAN_POINT('Ctrl Pts',(261.754727069591,78.2999231643027,230.397499740681));
#21017=CARTESIAN_POINT('Ctrl Pts',(263.533654545715,78.3947691062589,230.197080913061));
#21018=CARTESIAN_POINT('Ctrl Pts',(263.557302515181,77.8588297294342,228.466535359745));
#21019=CARTESIAN_POINT('Ctrl Pts',(261.949245797898,77.905077339807,230.518734113756));
#21020=CARTESIAN_POINT('Ctrl Pts',(263.538547887166,77.9742246260869,230.184893838673));
#21021=CARTESIAN_POINT('Ctrl Pts',(263.606591880382,77.3148820941748,228.695704330778));
#21022=CARTESIAN_POINT('Ctrl Pts',(262.433710331117,77.0716088320361,230.862258230087));
#21023=CARTESIAN_POINT('Ctrl Pts',(263.62457185023,77.0153725192018,230.390094211506));
#21024=CARTESIAN_POINT('Ctrl Pts',(263.755975405511,76.2858158960459,229.333149475148));
#21025=CARTESIAN_POINT('Ctrl Pts',(262.711999049712,76.651982580077,231.07693973435));
#21026=CARTESIAN_POINT('Ctrl Pts',(263.698661733633,76.5115820479241,230.587426418292));
#21027=CARTESIAN_POINT('Ctrl Pts',(263.852404590493,75.8249982256616,229.727424668816));
#21028=CARTESIAN_POINT('Ctrl Pts',(263.151909041546,75.9871679741599,231.451683298859));
#21029=CARTESIAN_POINT('Ctrl Pts',(263.858168373587,75.7622723596515,231.014329531148));
#21030=CARTESIAN_POINT('Ctrl Pts',(264.014706007827,75.1891126872917,230.390979291267));
#21031=CARTESIAN_POINT('Ctrl Pts',(263.302835955366,75.7588393827039,231.586229920659));
#21032=CARTESIAN_POINT('Ctrl Pts',(263.917768744924,75.5167006386232,231.174220647959));
#21033=CARTESIAN_POINT('Ctrl Pts',(264.072112191274,74.9857513363428,230.625585659508));
#21034=CARTESIAN_POINT('Ctrl Pts',(263.603229270728,75.2913050055119,231.871484249179));
#21035=CARTESIAN_POINT('Ctrl Pts',(264.048271575524,75.0381564136451,231.523754885091));
#21036=CARTESIAN_POINT('Ctrl Pts',(264.190557682095,74.5984025565875,231.111812803299));
#21037=CARTESIAN_POINT('Ctrl Pts',(263.752412397553,75.0525305312736,232.021888703375));
#21038=CARTESIAN_POINT('Ctrl Pts',(264.119123197883,74.8037832321443,231.713284495735));
#21039=CARTESIAN_POINT('Ctrl Pts',(264.251478238827,74.4146529473821,231.362943463785));
#21040=CARTESIAN_POINT('Ctrl Pts',(264.18801223314,74.318663255928,232.498072233561));
#21041=CARTESIAN_POINT('Ctrl Pts',(264.343108315152,74.1265992211969,232.310088246099));
#21042=CARTESIAN_POINT('Ctrl Pts',(264.437749904701,73.8878858377892,232.136325187552));
#21043=CARTESIAN_POINT('Ctrl Pts',(264.462022086343,73.805063319091,232.848874208672));
#21044=CARTESIAN_POINT('Ctrl Pts',(264.514363032579,73.6868688639842,232.764079118951));
#21045=CARTESIAN_POINT('Ctrl Pts',(264.566427694476,73.5692983043056,232.678673032712));
#21046=CARTESIAN_POINT('Ctrl Pts',(264.697446473732,73.2734363771458,233.239531522425));
#21047=CARTESIAN_POINT('Ctrl Pts',(264.697446473732,73.2734363771458,233.239531522425));
#21048=CARTESIAN_POINT('Ctrl Pts',(264.697446473732,73.2734363771458,233.239531522425));
#21049=CARTESIAN_POINT('Origin',(261.544965371427,78.4005022217613,228.365981599697));
#21050=CARTESIAN_POINT('Ctrl Pts',(269.854275011351,91.6534391605604,232.857577006965));
#21051=CARTESIAN_POINT('Ctrl Pts',(270.570059236857,90.5960147688002,232.385774045372));
#21052=CARTESIAN_POINT('Ctrl Pts',(270.968300873754,90.7966556084582,231.099602120239));
#21053=CARTESIAN_POINT('Ctrl Pts',(268.604744603454,91.0863950856132,232.405463537209));
#21054=CARTESIAN_POINT('Ctrl Pts',(269.432630245025,89.9764222651554,231.966890092694));
#21055=CARTESIAN_POINT('Ctrl Pts',(269.865690073407,90.2412177466641,230.608113673404));
#21056=CARTESIAN_POINT('Ctrl Pts',(267.464189276692,90.3711900279631,231.954019100255));
#21057=CARTESIAN_POINT('Ctrl Pts',(268.441024770316,89.2277365749088,231.570841083931));
#21058=CARTESIAN_POINT('Ctrl Pts',(268.856210587267,89.5480198264324,230.117467754446));
#21059=CARTESIAN_POINT('Ctrl Pts',(266.167696989619,89.2769186281834,231.44356147555));
#21060=CARTESIAN_POINT('Ctrl Pts',(267.355974305096,88.1615081899221,231.147215204369));
#21061=CARTESIAN_POINT('Ctrl Pts',(267.70390220799,88.49475462708,229.56261847886));
#21062=CARTESIAN_POINT('Ctrl Pts',(265.916094587479,89.0487894564945,231.344572511768));
#21063=CARTESIAN_POINT('Ctrl Pts',(267.143553518795,87.9376690682908,231.064711755392));
#21064=CARTESIAN_POINT('Ctrl Pts',(267.480019289714,88.2754841698382,229.45502105674));
#21065=CARTESIAN_POINT('Ctrl Pts',(265.4323791966,88.5772761662469,231.155524737661));
#21066=CARTESIAN_POINT('Ctrl Pts',(266.737690630021,87.4799990631403,230.908816464417));
#21067=CARTESIAN_POINT('Ctrl Pts',(267.049049592436,87.8228826485866,229.249532939607));
#21068=CARTESIAN_POINT('Ctrl Pts',(265.199425076782,88.3332231180283,231.065132840242));
#21069=CARTESIAN_POINT('Ctrl Pts',(266.543832749098,87.2455062460305,230.835276501227));
#21070=CARTESIAN_POINT('Ctrl Pts',(266.841215893656,87.588906918953,229.151280183409));
#21071=CARTESIAN_POINT('Ctrl Pts',(264.751404757504,87.8281195778466,230.893641171869));
#21072=CARTESIAN_POINT('Ctrl Pts',(266.173128968869,86.765355814543,230.697233263588));
#21073=CARTESIAN_POINT('Ctrl Pts',(266.440914797084,87.1052253190934,228.964874858366));
#21074=CARTESIAN_POINT('Ctrl Pts',(264.53633792299,87.5670701460064,230.812539697383));
#21075=CARTESIAN_POINT('Ctrl Pts',(265.99661567878,86.5197889764757,230.63287950567));
#21076=CARTESIAN_POINT('Ctrl Pts',(266.248446847576,86.8555204360023,228.876720429038));
#21077=CARTESIAN_POINT('Ctrl Pts',(264.124514799001,87.0272818564076,230.660721835472));
#21078=CARTESIAN_POINT('Ctrl Pts',(265.66024065455,86.0173256302242,230.513656268916));
#21079=CARTESIAN_POINT('Ctrl Pts',(265.879235516166,86.3397350702421,228.711699775841));
#21080=CARTESIAN_POINT('Ctrl Pts',(263.927191920059,86.7475695814584,230.58981851043));
#21081=CARTESIAN_POINT('Ctrl Pts',(265.500275599213,85.7597404016426,230.458803159134));
#21082=CARTESIAN_POINT('Ctrl Pts',(265.701980328563,86.0727273676906,228.634630347835));
#21083=CARTESIAN_POINT('Ctrl Pts',(263.371013260911,85.8919630165414,230.396915586166));
#21084=CARTESIAN_POINT('Ctrl Pts',(265.048852082573,84.9762036078638,230.310332484399));
#21085=CARTESIAN_POINT('Ctrl Pts',(265.201250579595,85.2567685807412,228.424951655098));
#21086=CARTESIAN_POINT('Ctrl Pts',(263.045775790527,85.2976453867214,230.293899870431));
#21087=CARTESIAN_POINT('Ctrl Pts',(264.789930470114,84.446363163279,230.234220035086));
#21088=CARTESIAN_POINT('Ctrl Pts',(264.906879405776,84.6910034207126,228.312977103783));
#21089=CARTESIAN_POINT('Ctrl Pts',(262.62687627125,84.3695387744554,230.181183241364));
#21090=CARTESIAN_POINT('Ctrl Pts',(264.453884252299,83.6314427756986,230.151510863018));
#21091=CARTESIAN_POINT('Ctrl Pts',(264.525038303666,83.808960737799,228.190457998417));
#21092=CARTESIAN_POINT('Ctrl Pts',(262.498781303485,84.0540433691424,230.150587542756));
#21093=CARTESIAN_POINT('Ctrl Pts',(264.35067673049,83.3559903592243,230.129269379279));
#21094=CARTESIAN_POINT('Ctrl Pts',(264.407749924432,83.5093611816478,228.157201521371));
#21095=CARTESIAN_POINT('Ctrl Pts',(262.26635036146,83.4103949526379,230.104064485338));
#21096=CARTESIAN_POINT('Ctrl Pts',(264.161522391596,82.7966223766408,230.095512210108));
#21097=CARTESIAN_POINT('Ctrl Pts',(264.193747582666,82.8986213128696,228.106632552918));
#21098=CARTESIAN_POINT('Ctrl Pts',(262.161617537659,83.0806079892046,230.088126104489));
#21099=CARTESIAN_POINT('Ctrl Pts',(264.075481010945,82.5118428801294,230.084054419952));
#21100=CARTESIAN_POINT('Ctrl Pts',(264.096659353448,82.5859337679919,228.089308076332));
#21101=CARTESIAN_POINT('Ctrl Pts',(261.888691546354,82.0869216485276,230.063791396278));
#21102=CARTESIAN_POINT('Ctrl Pts',(263.846724958899,81.6550061013845,230.066518035117));
#21103=CARTESIAN_POINT('Ctrl Pts',(263.841428021229,81.6444770955451,228.062857080858));
#21104=CARTESIAN_POINT('Ctrl Pts',(261.760569838213,81.4178671457201,230.078387323601));
#21105=CARTESIAN_POINT('Ctrl Pts',(263.733391992834,81.0841958360596,230.076835183321));
#21106=CARTESIAN_POINT('Ctrl Pts',(263.718253822345,81.0115115254556,228.078722362158));
#21107=CARTESIAN_POINT('Ctrl Pts',(261.60811471911,80.0651323652977,230.166713788174));
#21108=CARTESIAN_POINT('Ctrl Pts',(263.579114429171,79.9201348333107,230.140876788285));
#21109=CARTESIAN_POINT('Ctrl Pts',(263.562456729262,79.7335113896652,228.174730202189));
#21110=CARTESIAN_POINT('Ctrl Pts',(261.584153941217,79.3806125524342,230.240765568358));
#21111=CARTESIAN_POINT('Ctrl Pts',(263.538621025243,79.3309179399804,230.194359322608));
#21112=CARTESIAN_POINT('Ctrl Pts',(263.53014583648,79.0876936137149,228.255221557826));
#21113=CARTESIAN_POINT('Ctrl Pts',(261.613732932928,78.6920384763593,230.34343273927));
#21114=CARTESIAN_POINT('Ctrl Pts',(263.538324332359,78.7241922265802,230.271761815837));
#21115=CARTESIAN_POINT('Ctrl Pts',(263.544604216139,78.4389366559092,228.366817597905));
#21116=CARTESIAN_POINT('Origin',(126.004365242683,113.565857732007,235.454046952338));
#21117=CARTESIAN_POINT('Origin',(128.290003445999,123.478408390104,235.454046952333));
#21118=CARTESIAN_POINT('Origin',(123.718727039363,103.653307073912,235.454046952337));
#21119=CARTESIAN_POINT('Origin',(122.575907937704,98.6970317448653,244.263820043021));
#21120=CARTESIAN_POINT('Origin',(121.433088836045,93.7407564158189,253.073593133703));
#21121=CARTESIAN_POINT('Origin',(129.432822547662,128.434683719148,244.263820043021));
#21122=CARTESIAN_POINT('Origin',(130.575641649323,133.390959048194,253.073593133703));
#21123=CARTESIAN_POINT('Origin',(122.575907937704,98.6970317448653,261.883366224386));
#21124=CARTESIAN_POINT('Origin',(123.718727039364,103.653307073913,270.693139315068));
#21125=CARTESIAN_POINT('Origin',(129.432822547662,128.434683719148,261.883366224386));
#21126=CARTESIAN_POINT('Origin',(128.290003446003,123.4784083901,270.693139315068));
#21127=CARTESIAN_POINT('Origin',(126.004365242683,113.565857732007,270.693139315069));
#21128=CARTESIAN_POINT('Origin',(234.789304633949,166.98951318199,253.073593133703));
#27761=UNCERTAINTY_MEASURE_WITH_UNIT(LENGTH_MEASURE(0.01),#27808,
'DISTANCE_ACCURACY_VALUE',
'Maximum model space distance between geometric entities at asserted c
onnectivities');
#27778=UNCERTAINTY_MEASURE_WITH_UNIT(LENGTH_MEASURE(0.01),#27808,
'DISTANCE_ACCURACY_VALUE',
'Maximum model space distance between geometric entities at asserted c
onnectivities');
#27790=(
GEOMETRIC_REPRESENTATION_CONTEXT(3)
GLOBAL_UNCERTAINTY_ASSIGNED_CONTEXT((#27761))
GLOBAL_UNIT_ASSIGNED_CONTEXT((#27808,#27810,#27811))
REPRESENTATION_CONTEXT('','3D')
);
#27807=(
GEOMETRIC_REPRESENTATION_CONTEXT(3)
GLOBAL_UNCERTAINTY_ASSIGNED_CONTEXT((#27778))
GLOBAL_UNIT_ASSIGNED_CONTEXT((#27808,#27810,#27811))
REPRESENTATION_CONTEXT('','3D')
);
#27808=(
LENGTH_UNIT()
NAMED_UNIT(*)
SI_UNIT(.MILLI.,.METRE.)
);
#27810=(
NAMED_UNIT(*)
PLANE_ANGLE_UNIT()
SI_UNIT($,.RADIAN.)
);
#27811=(
NAMED_UNIT(*)
SI_UNIT($,.STERADIAN.)
SOLID_ANGLE_UNIT()
);
#27823=SHAPE_DEFINITION_REPRESENTATION(#27856,#27910);
#27856=PRODUCT_DEFINITION_SHAPE('',$,#27939);
#27910=SHAPE_REPRESENTATION('',(#12994),#27790);
#27927=PRODUCT_DEFINITION_CONTEXT('part definition',#28013,'design');
#27939=PRODUCT_DEFINITION('Pump Body','Pump Body',#27967,#27927);
#27967=PRODUCT_DEFINITION_FORMATION('',$,#28026);
#28013=APPLICATION_CONTEXT('Managed model based 3d engineering');
#28014=PRODUCT_CONTEXT('part definition',#28013,'mechanical');
#28026=PRODUCT('Pump Body','Pump Body',$,(#28014));
#28050=COLOUR_RGB('Dark Blue',0.08,0.2,0.34);
#28051=FILL_AREA_STYLE_COLOUR('',#28050);
#28052=FILL_AREA_STYLE('',(#28051));
#28053=SURFACE_STYLE_FILL_AREA(#28052);
#28054=SURFACE_SIDE_STYLE('',(#28053));
#28055=SURFACE_STYLE_USAGE(.BOTH.,#28054);
#28056=PRESENTATION_STYLE_ASSIGNMENT((#28055));
ENDSEC;
END-ISO-10303-21;
